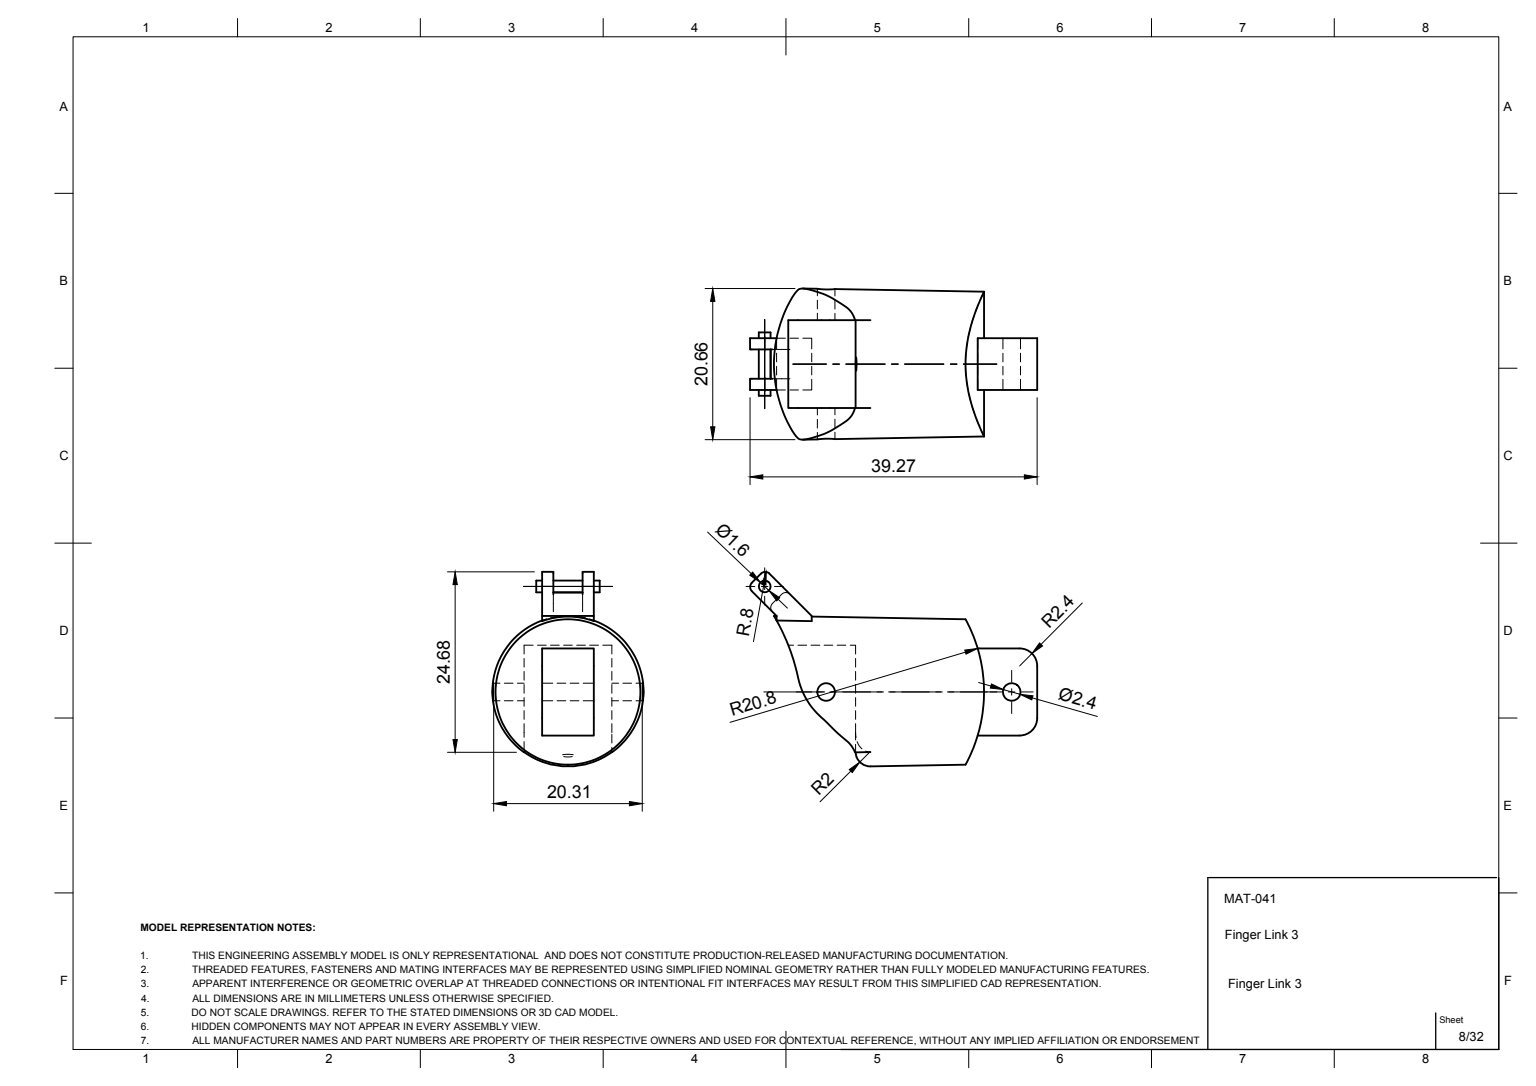
ISO-10303-21;
HEADER;
/* Generated by software containing ST-Developer
 * from STEP Tools, Inc. (www.steptools.com) 
 */

FILE_DESCRIPTION(
/* description */ ('STEP AP214'),
/* implementation_level */ '2;1');

FILE_NAME(
/* name */ 'Finger Link 3.step',
/* time_stamp */ '2026-11-14T21:57:47-08:00',
/* author */ (''),
/* organization */ (''),
/* preprocessor_version */ 'ST-DEVELOPER v20.2',
/* originating_system */ 'Autodesk Translation Framework v15.17.0.0',
/* authorisation */ '');

FILE_SCHEMA (('AUTOMOTIVE_DESIGN { 1 0 10303 214 3 1 1 }'));
ENDSEC;

DATA;
#10=MECHANICAL_DESIGN_GEOMETRIC_PRESENTATION_REPRESENTATION('',(#251),#13199);
#121=CONICAL_SURFACE('',#7376,10.4,0.0174532925199433);
#122=CONICAL_SURFACE('',#7390,10.4,0.0174532925199433);
#160=B_SPLINE_CURVE_WITH_KNOTS('',3,(#11078,#11079,#11080,#11081,#11082,
#11083,#11084,#11085,#11086,#11087,#11088,#11089,#11090,#11091,#11092,#11093,
#11094,#11095),.UNSPECIFIED.,.F.,.F.,(4,2,2,2,2,2,2,2,4),(0.904679564012803,
0.949860863856685,0.995042163700566,1.04019902886361,1.08535589402665,1.13069343457465,
1.17603097512264,1.22135607806746,1.26668118101228),.UNSPECIFIED.);
#161=B_SPLINE_CURVE_WITH_KNOTS('',3,(#11096,#11097,#11098,#11099,#11100,
#11101,#11102,#11103,#11104,#11105,#11106,#11107,#11108,#11109,#11110,#11111,
#11112,#11113,#11114),.UNSPECIFIED.,.F.,.F.,(4,2,2,2,3,2,2,2,4),(0.542677947013326,
0.588003049958145,0.633328152902964,0.678665693450959,0.724003233998953,
0.769160099161996,0.814316964325039,0.859498264168921,0.904679564012803),
 .UNSPECIFIED.);
#162=B_SPLINE_CURVE_WITH_KNOTS('',3,(#11118,#11119,#11120,#11121,#11122,
#11123,#11124,#11125,#11126,#11127,#11128,#11129,#11130,#11131,#11132,#11133,
#11134,#11135),.UNSPECIFIED.,.F.,.F.,(4,2,2,2,2,2,2,2,4),(-0.542677947013326,
-0.497352844068507,-0.452027741123688,-0.406690200575693,-0.361352660027699,
-0.316195794864656,-0.271038929701613,-0.225857629857731,-0.180676330013849),
 .UNSPECIFIED.);
#163=B_SPLINE_CURVE_WITH_KNOTS('',3,(#11139,#11140,#11141,#11142,#11143,
#11144,#11145,#11146,#11147,#11148,#11149,#11150,#11151,#11152,#11153,#11154,
#11155,#11156,#11157),.UNSPECIFIED.,.F.,.F.,(4,2,2,2,3,2,2,2,4),(-0.180676330013849,
-0.135495030169968,-0.0903137303260857,-0.0451568651630429,0.,0.0453375405479944,
0.0906750810959889,0.136000184040808,0.181325286985627),.UNSPECIFIED.);
#164=B_SPLINE_CURVE_WITH_KNOTS('',3,(#11163,#11164,#11165,#11166),
 .UNSPECIFIED.,.F.,.F.,(4,4),(0.0291654849228324,0.031266531407063),
 .UNSPECIFIED.);
#165=B_SPLINE_CURVE_WITH_KNOTS('',3,(#11168,#11169,#11170,#11171,#11172,
#11173,#11174,#11175),.UNSPECIFIED.,.F.,.F.,(4,2,2,4),(0.276435365996458,
0.375879882596353,0.487798645153617,0.537259984529731),.UNSPECIFIED.);
#166=B_SPLINE_CURVE_WITH_KNOTS('',3,(#11177,#11178,#11179,#11180),
 .UNSPECIFIED.,.F.,.F.,(4,4),(1.06524753198133,1.38156085898599),
 .UNSPECIFIED.);
#167=B_SPLINE_CURVE_WITH_KNOTS('',3,(#11182,#11183,#11184,#11185,#11186,
#11187),.UNSPECIFIED.,.F.,.F.,(4,2,4),(1.75246957687291,1.78785142251735,
1.90812306822259),.UNSPECIFIED.);
#168=B_SPLINE_CURVE_WITH_KNOTS('',3,(#11189,#11190,#11191,#11192,#11193,
#11194,#11195,#11196,#11197,#11198),.UNSPECIFIED.,.F.,.F.,(4,2,2,2,4),(5.98774864501298,
5.99007118193337,6.16584174870578,6.34161231547819,6.60463416407235),
 .UNSPECIFIED.);
#169=B_SPLINE_CURVE_WITH_KNOTS('',3,(#11200,#11201,#11202,#11203,#11204,
#11205,#11206,#11207,#11208,#11209),.UNSPECIFIED.,.F.,.F.,(4,2,2,2,4),(3.5239413534678,
3.56975642433501,3.96700634430097,4.37440770292553,4.58682119202782),
 .UNSPECIFIED.);
#170=B_SPLINE_CURVE_WITH_KNOTS('',3,(#11211,#11212,#11213,#11214,#11215,
#11216,#11217),.UNSPECIFIED.,.F.,.F.,(4,3,4),(0.0179093691038515,0.0203472114171927,
0.0227101968893206),.UNSPECIFIED.);
#171=B_SPLINE_CURVE_WITH_KNOTS('',3,(#11223,#11224,#11225,#11226,#11227,
#11228,#11229,#11230,#11231,#11232,#11233,#11234,#11235,#11236,#11237,#11238,
#11239,#11240),.UNSPECIFIED.,.F.,.F.,(4,2,2,2,2,2,2,2,4),(3.04488517957055,
3.42615346027245,3.80742174097434,4.18737194191896,4.56732214286358,4.94727660886795,
5.32723107487233,5.70850071700671,6.08977035914109),.UNSPECIFIED.);
#172=B_SPLINE_CURVE_WITH_KNOTS('',3,(#11241,#11242,#11243,#11244,#11245,
#11246,#11247,#11248,#11249,#11250,#11251,#11252,#11253,#11254,#11255,#11256,
#11257,#11258),.UNSPECIFIED.,.F.,.F.,(4,2,2,2,2,2,2,2,4),(0.,0.381269642134383,
0.762539284268766,1.14249375027314,1.52244821627752,1.90239841722213,2.28234861816675,
2.66361689886865,3.04488517957055),.UNSPECIFIED.);
#173=B_SPLINE_CURVE_WITH_KNOTS('',3,(#11262,#11263,#11264,#11265,#11266,
#11267,#11268),.UNSPECIFIED.,.F.,.F.,(4,3,4),(0.0179842259481975,0.0203472114199994,
0.0227850537330044),.UNSPECIFIED.);
#174=B_SPLINE_CURVE_WITH_KNOTS('',3,(#11270,#11271,#11272,#11273,#11274,
#11275,#11276,#11277,#11278,#11279),.UNSPECIFIED.,.F.,.F.,(4,2,2,2,4),(1.75819181671029,
1.97060530581257,2.37800666443714,2.7752565844031,2.82107165527031),
 .UNSPECIFIED.);
#175=B_SPLINE_CURVE_WITH_KNOTS('',3,(#11281,#11282,#11283,#11284,#11285,
#11286,#11287,#11288,#11289,#11290),.UNSPECIFIED.,.F.,.F.,(4,2,2,2,4),(9.36812303237173,
9.63114488096588,9.80691544773829,9.9826860145107,9.98500855143109),
 .UNSPECIFIED.);
#176=B_SPLINE_CURVE_WITH_KNOTS('',3,(#11292,#11293,#11294,#11295,#11296,
#11297),.UNSPECIFIED.,.F.,.F.,(4,2,4),(4.24121592260514,4.36148756831038,
4.39686941395482),.UNSPECIFIED.);
#177=B_SPLINE_CURVE_WITH_KNOTS('',3,(#11299,#11300,#11301,#11302),
 .UNSPECIFIED.,.F.,.F.,(4,4),(5.68043931343762,5.99675264044228),
 .UNSPECIFIED.);
#178=B_SPLINE_CURVE_WITH_KNOTS('',3,(#11304,#11305,#11306,#11307,#11308,
#11309,#11310,#11311),.UNSPECIFIED.,.F.,.F.,(4,2,2,4),(1.76236608590955,
1.81182742528566,1.92374618784292,2.02319070444282),.UNSPECIFIED.);
#179=B_SPLINE_CURVE_WITH_KNOTS('',3,(#11312,#11313,#11314,#11315),
 .UNSPECIFIED.,.F.,.F.,(4,4),(0.0094623862109046,0.0115634326876449),
 .UNSPECIFIED.);
#180=B_SPLINE_CURVE_WITH_KNOTS('',3,(#11332,#11333,#11334,#11335,#11336,
#11337,#11338,#11339,#11340,#11341,#11342,#11343,#11344),.UNSPECIFIED.,
 .F.,.F.,(4,3,2,2,2,4),(1.6015262701395,1.6049878447796,1.6729249721852,
1.74884321655348,1.83898176381711,1.95424158697802),.UNSPECIFIED.);
#181=B_SPLINE_CURVE_WITH_KNOTS('',3,(#11345,#11346,#11347,#11348,#11349,
#11350,#11351,#11352,#11353,#11354,#11355,#11356,#11357),.UNSPECIFIED.,
 .F.,.F.,(4,2,2,2,3,4),(1.25494218036839,1.36265497339682,1.4481494572272,
1.53110216280993,1.60422001043371,1.60768158507379),.UNSPECIFIED.);
#182=B_SPLINE_CURVE_WITH_KNOTS('',3,(#11359,#11360,#11361,#11362,#11363,
#11364,#11365,#11366,#11367,#11368,#11369,#11370,#11371,#11372,#11373,#11374,
#11375,#11376,#11377,#11378,#11379,#11380,#11381,#11382,#11383,#11384,#11385,
#11386,#11387,#11388,#11389,#11390,#11391,#11392,#11393,#11394,#11395,#11396,
#11397,#11398,#11399,#11400,#11401,#11402,#11403,#11404,#11405,#11406,#11407,
#11408,#11409,#11410),.UNSPECIFIED.,.T.,.F.,(4,2,2,2,2,2,2,2,2,2,2,2,2,
2,2,2,2,2,2,2,2,2,2,2,2,4),(-0.41069396663975,-0.366983311744642,-0.333124597039194,
-0.316725158605419,-0.311400724276707,-0.308795794387217,-0.307003152587989,
-0.305253095176476,-0.302970204179655,-0.299167956861605,-0.28993505003161,
-0.264304988598304,-0.228809697804181,-0.190091960609317,-0.153364093718904,
-0.124905530199035,-0.112501594518716,-0.107965577825246,-0.105609428487505,
-0.103889729748576,-0.102119162499972,-0.0996651361174354,-0.0953267397354206,
-0.0781357693656503,-0.0445945135149615,0.),.UNSPECIFIED.);
#183=B_SPLINE_CURVE_WITH_KNOTS('',3,(#11416,#11417,#11418,#11419,#11420,
#11421),.UNSPECIFIED.,.F.,.F.,(4,2,4),(-3.5239413534678,-3.17250650436905,
-2.82107165527031),.UNSPECIFIED.);
#215=SHAPE_REPRESENTATION_RELATIONSHIP('SRR','None',#13283,#233);
#233=ADVANCED_BREP_SHAPE_REPRESENTATION('',(#269),#13179);
#251=STYLED_ITEM('',(#13409),#269);
#269=MANIFOLD_SOLID_BREP('Body1',#6846);
#312=FACE_BOUND('',#2374,.T.);
#313=FACE_BOUND('',#2375,.T.);
#314=FACE_BOUND('',#2379,.T.);
#315=FACE_BOUND('',#2384,.T.);
#316=FACE_BOUND('',#2387,.T.);
#317=FACE_BOUND('',#2389,.T.);
#318=FACE_BOUND('',#2393,.T.);
#319=FACE_BOUND('',#2396,.T.);
#320=FACE_BOUND('',#2402,.T.);
#321=FACE_BOUND('',#2404,.T.);
#322=FACE_BOUND('',#2415,.T.);
#323=FACE_BOUND('',#2418,.T.);
#463=PLANE('',#7389);
#464=PLANE('',#7395);
#465=PLANE('',#7396);
#466=PLANE('',#7400);
#467=PLANE('',#7404);
#468=PLANE('',#7405);
#469=PLANE('',#7406);
#470=PLANE('',#7409);
#471=PLANE('',#7410);
#472=PLANE('',#7413);
#473=PLANE('',#7414);
#474=PLANE('',#7415);
#475=PLANE('',#7416);
#476=PLANE('',#7417);
#477=PLANE('',#7422);
#478=PLANE('',#7427);
#479=PLANE('',#7428);
#480=PLANE('',#7435);
#481=PLANE('',#7436);
#482=PLANE('',#7439);
#483=PLANE('',#7440);
#484=PLANE('',#7443);
#795=LINE('',#11052,#1313);
#796=LINE('',#11058,#1314);
#797=LINE('',#11064,#1315);
#798=LINE('',#11070,#1316);
#799=LINE('',#11076,#1317);
#800=LINE('',#11137,#1318);
#801=LINE('',#11221,#1319);
#802=LINE('',#11318,#1320);
#803=LINE('',#11321,#1321);
#804=LINE('',#11326,#1322);
#805=LINE('',#11327,#1323);
#806=LINE('',#11415,#1324);
#807=LINE('',#11423,#1325);
#808=LINE('',#11426,#1326);
#809=LINE('',#11430,#1327);
#810=LINE('',#11432,#1328);
#811=LINE('',#11434,#1329);
#812=LINE('',#11435,#1330);
#813=LINE('',#11441,#1331);
#814=LINE('',#11445,#1332);
#815=LINE('',#11449,#1333);
#816=LINE('',#11451,#1334);
#817=LINE('',#11452,#1335);
#818=LINE('',#11458,#1336);
#819=LINE('',#11463,#1337);
#820=LINE('',#11468,#1338);
#821=LINE('',#11470,#1339);
#822=LINE('',#11471,#1340);
#823=LINE('',#11475,#1341);
#824=LINE('',#11479,#1342);
#825=LINE('',#11480,#1343);
#826=LINE('',#11482,#1344);
#827=LINE('',#11486,#1345);
#828=LINE('',#11487,#1346);
#829=LINE('',#11490,#1347);
#830=LINE('',#11494,#1348);
#831=LINE('',#11497,#1349);
#832=LINE('',#11499,#1350);
#833=LINE('',#11501,#1351);
#834=LINE('',#11503,#1352);
#835=LINE('',#11504,#1353);
#836=LINE('',#11508,#1354);
#837=LINE('',#11510,#1355);
#838=LINE('',#11512,#1356);
#839=LINE('',#11513,#1357);
#840=LINE('',#11514,#1358);
#841=LINE('',#11518,#1359);
#842=LINE('',#11519,#1360);
#843=LINE('',#11520,#1361);
#844=LINE('',#11524,#1362);
#845=LINE('',#11526,#1363);
#846=LINE('',#11528,#1364);
#847=LINE('',#11529,#1365);
#848=LINE('',#11551,#1366);
#849=LINE('',#11553,#1367);
#850=LINE('',#11555,#1368);
#851=LINE('',#11556,#1369);
#852=LINE('',#11559,#1370);
#853=LINE('',#11563,#1371);
#854=LINE('',#11566,#1372);
#855=LINE('',#11567,#1373);
#856=LINE('',#11571,#1374);
#857=LINE('',#11574,#1375);
#858=LINE('',#11581,#1376);
#859=LINE('',#11583,#1377);
#1313=VECTOR('',#8618,1.2);
#1314=VECTOR('',#8625,0.800000000000001);
#1315=VECTOR('',#8632,0.800000000000001);
#1316=VECTOR('',#8639,0.800000000000001);
#1317=VECTOR('',#8646,1.2);
#1318=VECTOR('',#8649,1.2);
#1319=VECTOR('',#8658,10.4);
#1320=VECTOR('',#8663,1000.);
#1321=VECTOR('',#8666,1000.);
#1322=VECTOR('',#8671,1000.);
#1323=VECTOR('',#8672,1000.);
#1324=VECTOR('',#8681,1000.);
#1325=VECTOR('',#8682,1000.);
#1326=VECTOR('',#8685,1000.);
#1327=VECTOR('',#8688,1000.);
#1328=VECTOR('',#8689,1000.);
#1329=VECTOR('',#8690,1000.);
#1330=VECTOR('',#8691,1000.);
#1331=VECTOR('',#8698,1000.);
#1332=VECTOR('',#8701,1000.);
#1333=VECTOR('',#8706,1000.);
#1334=VECTOR('',#8707,1000.);
#1335=VECTOR('',#8708,1000.);
#1336=VECTOR('',#8717,1000.);
#1337=VECTOR('',#8724,1000.);
#1338=VECTOR('',#8731,1000.);
#1339=VECTOR('',#8732,1000.);
#1340=VECTOR('',#8733,1000.);
#1341=VECTOR('',#8736,1000.);
#1342=VECTOR('',#8739,1000.);
#1343=VECTOR('',#8740,1000.);
#1344=VECTOR('',#8741,1000.);
#1345=VECTOR('',#8746,1000.);
#1346=VECTOR('',#8747,1000.);
#1347=VECTOR('',#8750,1000.);
#1348=VECTOR('',#8755,1000.);
#1349=VECTOR('',#8758,1000.);
#1350=VECTOR('',#8759,1000.);
#1351=VECTOR('',#8760,1000.);
#1352=VECTOR('',#8761,1000.);
#1353=VECTOR('',#8762,1000.);
#1354=VECTOR('',#8765,1000.);
#1355=VECTOR('',#8766,1000.);
#1356=VECTOR('',#8767,1000.);
#1357=VECTOR('',#8768,1000.);
#1358=VECTOR('',#8769,1000.);
#1359=VECTOR('',#8772,1000.);
#1360=VECTOR('',#8773,1000.);
#1361=VECTOR('',#8774,1000.);
#1362=VECTOR('',#8777,1000.);
#1363=VECTOR('',#8778,1000.);
#1364=VECTOR('',#8779,1000.);
#1365=VECTOR('',#8780,1000.);
#1366=VECTOR('',#8819,1000.);
#1367=VECTOR('',#8820,1000.);
#1368=VECTOR('',#8821,1000.);
#1369=VECTOR('',#8822,1000.);
#1370=VECTOR('',#8825,1000.);
#1371=VECTOR('',#8830,1000.);
#1372=VECTOR('',#8833,1000.);
#1373=VECTOR('',#8834,1000.);
#1374=VECTOR('',#8839,1000.);
#1375=VECTOR('',#8844,1000.);
#1376=VECTOR('',#8857,1000.);
#1377=VECTOR('',#8860,1000.);
#1705=CYLINDRICAL_SURFACE('',#7360,1.2);
#1706=CYLINDRICAL_SURFACE('',#7363,0.800000000000001);
#1707=CYLINDRICAL_SURFACE('',#7366,0.800000000000001);
#1708=CYLINDRICAL_SURFACE('',#7369,0.800000000000001);
#1709=CYLINDRICAL_SURFACE('',#7372,1.2);
#1710=CYLINDRICAL_SURFACE('',#7374,1.2);
#1711=CYLINDRICAL_SURFACE('',#7380,16.7532667406203);
#1712=CYLINDRICAL_SURFACE('',#7382,16.7532667406203);
#1713=CYLINDRICAL_SURFACE('',#7386,28.);
#1714=CYLINDRICAL_SURFACE('',#7392,20.8);
#1715=CYLINDRICAL_SURFACE('',#7429,0.8);
#1716=CYLINDRICAL_SURFACE('',#7430,0.8);
#1717=CYLINDRICAL_SURFACE('',#7431,0.8);
#1718=CYLINDRICAL_SURFACE('',#7432,0.8);
#1719=CYLINDRICAL_SURFACE('',#7433,0.8);
#1720=CYLINDRICAL_SURFACE('',#7434,0.8);
#1721=CYLINDRICAL_SURFACE('',#7444,2.4);
#1722=CYLINDRICAL_SURFACE('',#7445,2.4);
#1723=CYLINDRICAL_SURFACE('',#7446,10.);
#1724=CYLINDRICAL_SURFACE('',#7447,10.);
#1725=CYLINDRICAL_SURFACE('',#7448,4.06015460582196);
#1726=CYLINDRICAL_SURFACE('',#7449,4.06015460582196);
#1727=CYLINDRICAL_SURFACE('',#7450,4.06015460582196);
#1728=CYLINDRICAL_SURFACE('',#7451,22.);
#1729=CYLINDRICAL_SURFACE('',#7452,22.);
#1948=FACE_OUTER_BOUND('',#2367,.T.);
#1949=FACE_OUTER_BOUND('',#2368,.T.);
#1950=FACE_OUTER_BOUND('',#2369,.T.);
#1951=FACE_OUTER_BOUND('',#2370,.T.);
#1952=FACE_OUTER_BOUND('',#2371,.T.);
#1953=FACE_OUTER_BOUND('',#2372,.T.);
#1954=FACE_OUTER_BOUND('',#2373,.T.);
#1955=FACE_OUTER_BOUND('',#2376,.T.);
#1956=FACE_OUTER_BOUND('',#2377,.T.);
#1957=FACE_OUTER_BOUND('',#2378,.T.);
#1958=FACE_OUTER_BOUND('',#2380,.T.);
#1959=FACE_OUTER_BOUND('',#2381,.T.);
#1960=FACE_OUTER_BOUND('',#2382,.T.);
#1961=FACE_OUTER_BOUND('',#2383,.T.);
#1962=FACE_OUTER_BOUND('',#2385,.T.);
#1963=FACE_OUTER_BOUND('',#2386,.T.);
#1964=FACE_OUTER_BOUND('',#2388,.T.);
#1965=FACE_OUTER_BOUND('',#2390,.T.);
#1966=FACE_OUTER_BOUND('',#2391,.T.);
#1967=FACE_OUTER_BOUND('',#2392,.T.);
#1968=FACE_OUTER_BOUND('',#2394,.T.);
#1969=FACE_OUTER_BOUND('',#2395,.T.);
#1970=FACE_OUTER_BOUND('',#2397,.T.);
#1971=FACE_OUTER_BOUND('',#2398,.T.);
#1972=FACE_OUTER_BOUND('',#2399,.T.);
#1973=FACE_OUTER_BOUND('',#2400,.T.);
#1974=FACE_OUTER_BOUND('',#2401,.T.);
#1975=FACE_OUTER_BOUND('',#2403,.T.);
#1976=FACE_OUTER_BOUND('',#2405,.T.);
#1977=FACE_OUTER_BOUND('',#2406,.T.);
#1978=FACE_OUTER_BOUND('',#2407,.T.);
#1979=FACE_OUTER_BOUND('',#2408,.T.);
#1980=FACE_OUTER_BOUND('',#2409,.T.);
#1981=FACE_OUTER_BOUND('',#2410,.T.);
#1982=FACE_OUTER_BOUND('',#2411,.T.);
#1983=FACE_OUTER_BOUND('',#2412,.T.);
#1984=FACE_OUTER_BOUND('',#2413,.T.);
#1985=FACE_OUTER_BOUND('',#2414,.T.);
#1986=FACE_OUTER_BOUND('',#2416,.T.);
#1987=FACE_OUTER_BOUND('',#2417,.T.);
#1988=FACE_OUTER_BOUND('',#2419,.T.);
#1989=FACE_OUTER_BOUND('',#2420,.T.);
#1990=FACE_OUTER_BOUND('',#2421,.T.);
#1991=FACE_OUTER_BOUND('',#2422,.T.);
#1992=FACE_OUTER_BOUND('',#2423,.T.);
#1993=FACE_OUTER_BOUND('',#2424,.T.);
#1994=FACE_OUTER_BOUND('',#2425,.T.);
#1995=FACE_OUTER_BOUND('',#2426,.T.);
#1996=FACE_OUTER_BOUND('',#2427,.T.);
#1997=FACE_OUTER_BOUND('',#2428,.T.);
#2367=EDGE_LOOP('',(#5286,#5287,#5288,#5289));
#2368=EDGE_LOOP('',(#5290,#5291,#5292,#5293));
#2369=EDGE_LOOP('',(#5294,#5295,#5296,#5297));
#2370=EDGE_LOOP('',(#5298,#5299,#5300,#5301));
#2371=EDGE_LOOP('',(#5302,#5303,#5304,#5305,#5306));
#2372=EDGE_LOOP('',(#5307,#5308,#5309,#5310,#5311));
#2373=EDGE_LOOP('',(#5312,#5313,#5314,#5315,#5316,#5317,#5318,#5319,#5320,
#5321,#5322,#5323,#5324,#5325,#5326,#5327,#5328,#5329,#5330,#5331,#5332));
#2374=EDGE_LOOP('',(#5333,#5334));
#2375=EDGE_LOOP('',(#5335,#5336));
#2376=EDGE_LOOP('',(#5337,#5338,#5339,#5340));
#2377=EDGE_LOOP('',(#5341,#5342,#5343,#5344));
#2378=EDGE_LOOP('',(#5345,#5346,#5347,#5348));
#2379=EDGE_LOOP('',(#5349));
#2380=EDGE_LOOP('',(#5350,#5351,#5352,#5353,#5354,#5355,#5356,#5357));
#2381=EDGE_LOOP('',(#5358,#5359,#5360,#5361));
#2382=EDGE_LOOP('',(#5362,#5363));
#2383=EDGE_LOOP('',(#5364,#5365));
#2384=EDGE_LOOP('',(#5366,#5367,#5368,#5369));
#2385=EDGE_LOOP('',(#5370,#5371,#5372,#5373));
#2386=EDGE_LOOP('',(#5374,#5375,#5376,#5377,#5378,#5379,#5380,#5381,#5382));
#2387=EDGE_LOOP('',(#5383));
#2388=EDGE_LOOP('',(#5384,#5385,#5386,#5387,#5388,#5389,#5390,#5391,#5392));
#2389=EDGE_LOOP('',(#5393));
#2390=EDGE_LOOP('',(#5394,#5395,#5396,#5397));
#2391=EDGE_LOOP('',(#5398,#5399,#5400,#5401));
#2392=EDGE_LOOP('',(#5402,#5403,#5404,#5405,#5406,#5407,#5408,#5409));
#2393=EDGE_LOOP('',(#5410));
#2394=EDGE_LOOP('',(#5411,#5412,#5413,#5414,#5415));
#2395=EDGE_LOOP('',(#5416,#5417,#5418,#5419,#5420,#5421,#5422,#5423));
#2396=EDGE_LOOP('',(#5424));
#2397=EDGE_LOOP('',(#5425,#5426,#5427,#5428,#5429,#5430,#5431,#5432));
#2398=EDGE_LOOP('',(#5433,#5434,#5435,#5436,#5437,#5438,#5439,#5440));
#2399=EDGE_LOOP('',(#5441,#5442,#5443,#5444));
#2400=EDGE_LOOP('',(#5445,#5446,#5447,#5448));
#2401=EDGE_LOOP('',(#5449,#5450,#5451,#5452,#5453,#5454,#5455,#5456));
#2402=EDGE_LOOP('',(#5457));
#2403=EDGE_LOOP('',(#5458,#5459,#5460,#5461,#5462,#5463,#5464,#5465));
#2404=EDGE_LOOP('',(#5466));
#2405=EDGE_LOOP('',(#5467));
#2406=EDGE_LOOP('',(#5468));
#2407=EDGE_LOOP('',(#5469,#5470,#5471,#5472));
#2408=EDGE_LOOP('',(#5473,#5474,#5475,#5476));
#2409=EDGE_LOOP('',(#5477,#5478,#5479,#5480));
#2410=EDGE_LOOP('',(#5481,#5482,#5483,#5484));
#2411=EDGE_LOOP('',(#5485,#5486,#5487,#5488));
#2412=EDGE_LOOP('',(#5489,#5490,#5491,#5492));
#2413=EDGE_LOOP('',(#5493,#5494,#5495,#5496));
#2414=EDGE_LOOP('',(#5497,#5498,#5499,#5500,#5501,#5502));
#2415=EDGE_LOOP('',(#5503));
#2416=EDGE_LOOP('',(#5504,#5505,#5506,#5507));
#2417=EDGE_LOOP('',(#5508,#5509,#5510,#5511,#5512,#5513));
#2418=EDGE_LOOP('',(#5514));
#2419=EDGE_LOOP('',(#5515,#5516,#5517,#5518));
#2420=EDGE_LOOP('',(#5519,#5520,#5521,#5522));
#2421=EDGE_LOOP('',(#5523,#5524,#5525,#5526));
#2422=EDGE_LOOP('',(#5527,#5528,#5529,#5530));
#2423=EDGE_LOOP('',(#5531,#5532,#5533,#5534));
#2424=EDGE_LOOP('',(#5535));
#2425=EDGE_LOOP('',(#5536,#5537,#5538));
#2426=EDGE_LOOP('',(#5539,#5540,#5541));
#2427=EDGE_LOOP('',(#5542,#5543,#5544,#5545));
#2428=EDGE_LOOP('',(#5546,#5547,#5548,#5549));
#2818=CIRCLE('',#7361,1.2);
#2819=CIRCLE('',#7362,1.2);
#2820=CIRCLE('',#7364,0.800000000000001);
#2821=CIRCLE('',#7365,0.800000000000001);
#2822=CIRCLE('',#7367,0.800000000000001);
#2823=CIRCLE('',#7368,0.800000000000001);
#2824=CIRCLE('',#7370,0.800000000000001);
#2825=CIRCLE('',#7371,0.800000000000001);
#2826=CIRCLE('',#7373,1.2);
#2827=CIRCLE('',#7375,1.2);
#2828=CIRCLE('',#7377,10.169681257704);
#2829=CIRCLE('',#7378,10.3099206524828);
#2830=CIRCLE('',#7379,10.3099206524828);
#2831=CIRCLE('',#7381,16.7532667406203);
#2832=CIRCLE('',#7383,16.7532667406203);
#2833=CIRCLE('',#7385,8.16998586739121);
#2834=CIRCLE('',#7387,28.);
#2835=CIRCLE('',#7388,28.);
#2836=CIRCLE('',#7391,10.3937049641382);
#2837=CIRCLE('',#7393,20.8);
#2838=CIRCLE('',#7394,20.8);
#2839=CIRCLE('',#7397,4.06015460582196);
#2840=CIRCLE('',#7398,22.);
#2841=CIRCLE('',#7399,10.);
#2842=CIRCLE('',#7401,22.);
#2843=CIRCLE('',#7402,4.06015460582196);
#2844=CIRCLE('',#7403,10.);
#2845=CIRCLE('',#7407,0.8);
#2846=CIRCLE('',#7408,0.8);
#2847=CIRCLE('',#7411,0.8);
#2848=CIRCLE('',#7412,0.8);
#2849=CIRCLE('',#7418,0.8);
#2850=CIRCLE('',#7419,0.8);
#2851=CIRCLE('',#7420,0.8);
#2852=CIRCLE('',#7421,0.8);
#2853=CIRCLE('',#7423,0.8);
#2854=CIRCLE('',#7424,0.8);
#2855=CIRCLE('',#7425,0.8);
#2856=CIRCLE('',#7426,0.8);
#2857=CIRCLE('',#7437,2.4);
#2858=CIRCLE('',#7438,2.4);
#2859=CIRCLE('',#7441,2.4);
#2860=CIRCLE('',#7442,2.4);
#3230=VERTEX_POINT('',#11049);
#3231=VERTEX_POINT('',#11051);
#3232=VERTEX_POINT('',#11055);
#3233=VERTEX_POINT('',#11057);
#3234=VERTEX_POINT('',#11061);
#3235=VERTEX_POINT('',#11063);
#3236=VERTEX_POINT('',#11067);
#3237=VERTEX_POINT('',#11069);
#3238=VERTEX_POINT('',#11073);
#3239=VERTEX_POINT('',#11075);
#3240=VERTEX_POINT('',#11077);
#3241=VERTEX_POINT('',#11116);
#3242=VERTEX_POINT('',#11117);
#3243=VERTEX_POINT('',#11136);
#3244=VERTEX_POINT('',#11159);
#3245=VERTEX_POINT('',#11160);
#3246=VERTEX_POINT('',#11162);
#3247=VERTEX_POINT('',#11167);
#3248=VERTEX_POINT('',#11176);
#3249=VERTEX_POINT('',#11181);
#3250=VERTEX_POINT('',#11188);
#3251=VERTEX_POINT('',#11199);
#3252=VERTEX_POINT('',#11210);
#3253=VERTEX_POINT('',#11218);
#3254=VERTEX_POINT('',#11220);
#3255=VERTEX_POINT('',#11222);
#3256=VERTEX_POINT('',#11259);
#3257=VERTEX_POINT('',#11261);
#3258=VERTEX_POINT('',#11269);
#3259=VERTEX_POINT('',#11280);
#3260=VERTEX_POINT('',#11291);
#3261=VERTEX_POINT('',#11298);
#3262=VERTEX_POINT('',#11303);
#3263=VERTEX_POINT('',#11317);
#3264=VERTEX_POINT('',#11319);
#3265=VERTEX_POINT('',#11323);
#3266=VERTEX_POINT('',#11324);
#3267=VERTEX_POINT('',#11329);
#3268=VERTEX_POINT('',#11330);
#3269=VERTEX_POINT('',#11358);
#3270=VERTEX_POINT('',#11412);
#3271=VERTEX_POINT('',#11413);
#3272=VERTEX_POINT('',#11422);
#3273=VERTEX_POINT('',#11424);
#3274=VERTEX_POINT('',#11428);
#3275=VERTEX_POINT('',#11429);
#3276=VERTEX_POINT('',#11431);
#3277=VERTEX_POINT('',#11433);
#3278=VERTEX_POINT('',#11439);
#3279=VERTEX_POINT('',#11440);
#3280=VERTEX_POINT('',#11442);
#3281=VERTEX_POINT('',#11444);
#3282=VERTEX_POINT('',#11448);
#3283=VERTEX_POINT('',#11450);
#3284=VERTEX_POINT('',#11454);
#3285=VERTEX_POINT('',#11460);
#3286=VERTEX_POINT('',#11467);
#3287=VERTEX_POINT('',#11469);
#3288=VERTEX_POINT('',#11473);
#3289=VERTEX_POINT('',#11474);
#3290=VERTEX_POINT('',#11476);
#3291=VERTEX_POINT('',#11478);
#3292=VERTEX_POINT('',#11481);
#3293=VERTEX_POINT('',#11485);
#3294=VERTEX_POINT('',#11489);
#3295=VERTEX_POINT('',#11492);
#3296=VERTEX_POINT('',#11496);
#3297=VERTEX_POINT('',#11498);
#3298=VERTEX_POINT('',#11500);
#3299=VERTEX_POINT('',#11502);
#3300=VERTEX_POINT('',#11506);
#3301=VERTEX_POINT('',#11507);
#3302=VERTEX_POINT('',#11509);
#3303=VERTEX_POINT('',#11511);
#3304=VERTEX_POINT('',#11516);
#3305=VERTEX_POINT('',#11517);
#3306=VERTEX_POINT('',#11522);
#3307=VERTEX_POINT('',#11523);
#3308=VERTEX_POINT('',#11525);
#3309=VERTEX_POINT('',#11527);
#3310=VERTEX_POINT('',#11549);
#3311=VERTEX_POINT('',#11550);
#3312=VERTEX_POINT('',#11552);
#3313=VERTEX_POINT('',#11554);
#3314=VERTEX_POINT('',#11558);
#3315=VERTEX_POINT('',#11561);
#3316=VERTEX_POINT('',#11565);
#3317=VERTEX_POINT('',#11570);
#3980=EDGE_CURVE('',#3230,#3230,#2818,.T.);
#3981=EDGE_CURVE('',#3230,#3231,#795,.T.);
#3982=EDGE_CURVE('',#3231,#3231,#2819,.T.);
#3983=EDGE_CURVE('',#3232,#3232,#2820,.T.);
#3984=EDGE_CURVE('',#3232,#3233,#796,.T.);
#3985=EDGE_CURVE('',#3233,#3233,#2821,.T.);
#3986=EDGE_CURVE('',#3234,#3234,#2822,.T.);
#3987=EDGE_CURVE('',#3234,#3235,#797,.T.);
#3988=EDGE_CURVE('',#3235,#3235,#2823,.T.);
#3989=EDGE_CURVE('',#3236,#3236,#2824,.T.);
#3990=EDGE_CURVE('',#3236,#3237,#798,.T.);
#3991=EDGE_CURVE('',#3237,#3237,#2825,.T.);
#3992=EDGE_CURVE('',#3238,#3238,#2826,.T.);
#3993=EDGE_CURVE('',#3238,#3239,#799,.T.);
#3994=EDGE_CURVE('',#3239,#3240,#160,.T.);
#3995=EDGE_CURVE('',#3240,#3239,#161,.T.);
#3996=EDGE_CURVE('',#3241,#3242,#162,.T.);
#3997=EDGE_CURVE('',#3242,#3243,#800,.T.);
#3998=EDGE_CURVE('',#3243,#3243,#2827,.T.);
#3999=EDGE_CURVE('',#3242,#3241,#163,.T.);
#4000=EDGE_CURVE('',#3244,#3245,#2828,.T.);
#4001=EDGE_CURVE('',#3246,#3245,#164,.T.);
#4002=EDGE_CURVE('',#3247,#3246,#165,.T.);
#4003=EDGE_CURVE('',#3247,#3248,#166,.T.);
#4004=EDGE_CURVE('',#3249,#3248,#167,.T.);
#4005=EDGE_CURVE('',#3249,#3250,#168,.T.);
#4006=EDGE_CURVE('',#3251,#3250,#169,.T.);
#4007=EDGE_CURVE('',#3251,#3252,#170,.T.);
#4008=EDGE_CURVE('',#3252,#3253,#2829,.T.);
#4009=EDGE_CURVE('',#3253,#3254,#801,.T.);
#4010=EDGE_CURVE('',#3254,#3255,#171,.T.);
#4011=EDGE_CURVE('',#3255,#3254,#172,.T.);
#4012=EDGE_CURVE('',#3253,#3256,#2830,.T.);
#4013=EDGE_CURVE('',#3256,#3257,#173,.T.);
#4014=EDGE_CURVE('',#3258,#3257,#174,.T.);
#4015=EDGE_CURVE('',#3258,#3259,#175,.T.);
#4016=EDGE_CURVE('',#3260,#3259,#176,.T.);
#4017=EDGE_CURVE('',#3260,#3261,#177,.T.);
#4018=EDGE_CURVE('',#3262,#3261,#178,.T.);
#4019=EDGE_CURVE('',#3244,#3262,#179,.T.);
#4020=EDGE_CURVE('',#3248,#3263,#802,.T.);
#4021=EDGE_CURVE('',#3264,#3263,#2831,.T.);
#4022=EDGE_CURVE('',#3264,#3249,#803,.T.);
#4023=EDGE_CURVE('',#3265,#3266,#2832,.T.);
#4024=EDGE_CURVE('',#3265,#3260,#804,.T.);
#4025=EDGE_CURVE('',#3259,#3266,#805,.T.);
#4026=EDGE_CURVE('',#3267,#3268,#2833,.T.);
#4027=EDGE_CURVE('',#3245,#3267,#180,.T.);
#4028=EDGE_CURVE('',#3268,#3244,#181,.T.);
#4029=EDGE_CURVE('',#3269,#3269,#182,.T.);
#4030=EDGE_CURVE('',#3270,#3271,#2834,.T.);
#4031=EDGE_CURVE('',#3271,#3258,#806,.T.);
#4032=EDGE_CURVE('',#3257,#3251,#183,.T.);
#4033=EDGE_CURVE('',#3250,#3272,#807,.T.);
#4034=EDGE_CURVE('',#3272,#3273,#2835,.T.);
#4035=EDGE_CURVE('',#3270,#3273,#808,.T.);
#4036=EDGE_CURVE('',#3274,#3275,#809,.T.);
#4037=EDGE_CURVE('',#3275,#3276,#810,.T.);
#4038=EDGE_CURVE('',#3277,#3276,#811,.T.);
#4039=EDGE_CURVE('',#3277,#3274,#812,.T.);
#4040=EDGE_CURVE('',#3257,#3251,#2836,.T.);
#4041=EDGE_CURVE('',#3278,#3279,#813,.T.);
#4042=EDGE_CURVE('',#3280,#3278,#2837,.T.);
#4043=EDGE_CURVE('',#3281,#3280,#814,.T.);
#4044=EDGE_CURVE('',#3279,#3281,#2838,.T.);
#4045=EDGE_CURVE('',#3268,#3282,#815,.T.);
#4046=EDGE_CURVE('',#3283,#3282,#816,.T.);
#4047=EDGE_CURVE('',#3267,#3283,#817,.T.);
#4048=EDGE_CURVE('',#3262,#3284,#2839,.T.);
#4049=EDGE_CURVE('',#3284,#3265,#2840,.T.);
#4050=EDGE_CURVE('',#3266,#3271,#2841,.T.);
#4051=EDGE_CURVE('',#3282,#3270,#818,.T.);
#4052=EDGE_CURVE('',#3263,#3285,#2842,.T.);
#4053=EDGE_CURVE('',#3285,#3246,#2843,.T.);
#4054=EDGE_CURVE('',#3273,#3283,#819,.T.);
#4055=EDGE_CURVE('',#3272,#3264,#2844,.T.);
#4056=EDGE_CURVE('',#3257,#3286,#820,.T.);
#4057=EDGE_CURVE('',#3286,#3287,#821,.T.);
#4058=EDGE_CURVE('',#3251,#3287,#822,.T.);
#4059=EDGE_CURVE('',#3288,#3289,#823,.T.);
#4060=EDGE_CURVE('',#3288,#3290,#2845,.T.);
#4061=EDGE_CURVE('',#3290,#3291,#824,.T.);
#4062=EDGE_CURVE('',#3252,#3291,#825,.T.);
#4063=EDGE_CURVE('',#3292,#3287,#826,.T.);
#4064=EDGE_CURVE('',#3292,#3289,#2846,.T.);
#4065=EDGE_CURVE('',#3291,#3293,#827,.T.);
#4066=EDGE_CURVE('',#3256,#3293,#828,.T.);
#4067=EDGE_CURVE('',#3294,#3293,#829,.T.);
#4068=EDGE_CURVE('',#3294,#3275,#2847,.T.);
#4069=EDGE_CURVE('',#3274,#3295,#2848,.T.);
#4070=EDGE_CURVE('',#3295,#3286,#830,.T.);
#4071=EDGE_CURVE('',#3295,#3296,#831,.T.);
#4072=EDGE_CURVE('',#3296,#3297,#832,.T.);
#4073=EDGE_CURVE('',#3297,#3298,#833,.T.);
#4074=EDGE_CURVE('',#3298,#3299,#834,.T.);
#4075=EDGE_CURVE('',#3299,#3292,#835,.T.);
#4076=EDGE_CURVE('',#3300,#3301,#836,.T.);
#4077=EDGE_CURVE('',#3300,#3302,#837,.T.);
#4078=EDGE_CURVE('',#3303,#3302,#838,.T.);
#4079=EDGE_CURVE('',#3303,#3294,#839,.T.);
#4080=EDGE_CURVE('',#3290,#3301,#840,.T.);
#4081=EDGE_CURVE('',#3304,#3305,#841,.T.);
#4082=EDGE_CURVE('',#3304,#3288,#842,.T.);
#4083=EDGE_CURVE('',#3289,#3305,#843,.T.);
#4084=EDGE_CURVE('',#3306,#3307,#844,.T.);
#4085=EDGE_CURVE('',#3307,#3308,#845,.T.);
#4086=EDGE_CURVE('',#3309,#3308,#846,.T.);
#4087=EDGE_CURVE('',#3309,#3306,#847,.T.);
#4088=EDGE_CURVE('',#3276,#3303,#2849,.T.);
#4089=EDGE_CURVE('',#3302,#3307,#2850,.T.);
#4090=EDGE_CURVE('',#3306,#3297,#2851,.T.);
#4091=EDGE_CURVE('',#3296,#3277,#2852,.T.);
#4092=EDGE_CURVE('',#3301,#3304,#2853,.T.);
#4093=EDGE_CURVE('',#3305,#3299,#2854,.T.);
#4094=EDGE_CURVE('',#3298,#3309,#2855,.T.);
#4095=EDGE_CURVE('',#3308,#3300,#2856,.T.);
#4096=EDGE_CURVE('',#3310,#3311,#848,.T.);
#4097=EDGE_CURVE('',#3311,#3312,#849,.T.);
#4098=EDGE_CURVE('',#3312,#3313,#850,.T.);
#4099=EDGE_CURVE('',#3313,#3310,#851,.T.);
#4100=EDGE_CURVE('',#3278,#3314,#852,.T.);
#4101=EDGE_CURVE('',#3314,#3311,#2857,.T.);
#4102=EDGE_CURVE('',#3310,#3315,#2858,.T.);
#4103=EDGE_CURVE('',#3280,#3315,#853,.T.);
#4104=EDGE_CURVE('',#3279,#3316,#854,.T.);
#4105=EDGE_CURVE('',#3316,#3314,#855,.T.);
#4106=EDGE_CURVE('',#3312,#3316,#2859,.T.);
#4107=EDGE_CURVE('',#3281,#3317,#856,.T.);
#4108=EDGE_CURVE('',#3317,#3313,#2860,.T.);
#4109=EDGE_CURVE('',#3315,#3317,#857,.T.);
#4110=EDGE_CURVE('',#3261,#3284,#858,.T.);
#4111=EDGE_CURVE('',#3285,#3247,#859,.T.);
#5286=ORIENTED_EDGE('',*,*,#3980,.T.);
#5287=ORIENTED_EDGE('',*,*,#3981,.T.);
#5288=ORIENTED_EDGE('',*,*,#3982,.T.);
#5289=ORIENTED_EDGE('',*,*,#3981,.F.);
#5290=ORIENTED_EDGE('',*,*,#3983,.T.);
#5291=ORIENTED_EDGE('',*,*,#3984,.T.);
#5292=ORIENTED_EDGE('',*,*,#3985,.T.);
#5293=ORIENTED_EDGE('',*,*,#3984,.F.);
#5294=ORIENTED_EDGE('',*,*,#3986,.T.);
#5295=ORIENTED_EDGE('',*,*,#3987,.T.);
#5296=ORIENTED_EDGE('',*,*,#3988,.F.);
#5297=ORIENTED_EDGE('',*,*,#3987,.F.);
#5298=ORIENTED_EDGE('',*,*,#3989,.T.);
#5299=ORIENTED_EDGE('',*,*,#3990,.T.);
#5300=ORIENTED_EDGE('',*,*,#3991,.T.);
#5301=ORIENTED_EDGE('',*,*,#3990,.F.);
#5302=ORIENTED_EDGE('',*,*,#3992,.F.);
#5303=ORIENTED_EDGE('',*,*,#3993,.T.);
#5304=ORIENTED_EDGE('',*,*,#3994,.T.);
#5305=ORIENTED_EDGE('',*,*,#3995,.T.);
#5306=ORIENTED_EDGE('',*,*,#3993,.F.);
#5307=ORIENTED_EDGE('',*,*,#3996,.T.);
#5308=ORIENTED_EDGE('',*,*,#3997,.T.);
#5309=ORIENTED_EDGE('',*,*,#3998,.F.);
#5310=ORIENTED_EDGE('',*,*,#3997,.F.);
#5311=ORIENTED_EDGE('',*,*,#3999,.T.);
#5312=ORIENTED_EDGE('',*,*,#4000,.T.);
#5313=ORIENTED_EDGE('',*,*,#4001,.F.);
#5314=ORIENTED_EDGE('',*,*,#4002,.F.);
#5315=ORIENTED_EDGE('',*,*,#4003,.T.);
#5316=ORIENTED_EDGE('',*,*,#4004,.F.);
#5317=ORIENTED_EDGE('',*,*,#4005,.T.);
#5318=ORIENTED_EDGE('',*,*,#4006,.F.);
#5319=ORIENTED_EDGE('',*,*,#4007,.T.);
#5320=ORIENTED_EDGE('',*,*,#4008,.T.);
#5321=ORIENTED_EDGE('',*,*,#4009,.T.);
#5322=ORIENTED_EDGE('',*,*,#4010,.T.);
#5323=ORIENTED_EDGE('',*,*,#4011,.T.);
#5324=ORIENTED_EDGE('',*,*,#4009,.F.);
#5325=ORIENTED_EDGE('',*,*,#4012,.T.);
#5326=ORIENTED_EDGE('',*,*,#4013,.T.);
#5327=ORIENTED_EDGE('',*,*,#4014,.F.);
#5328=ORIENTED_EDGE('',*,*,#4015,.T.);
#5329=ORIENTED_EDGE('',*,*,#4016,.F.);
#5330=ORIENTED_EDGE('',*,*,#4017,.T.);
#5331=ORIENTED_EDGE('',*,*,#4018,.F.);
#5332=ORIENTED_EDGE('',*,*,#4019,.F.);
#5333=ORIENTED_EDGE('',*,*,#3996,.F.);
#5334=ORIENTED_EDGE('',*,*,#3999,.F.);
#5335=ORIENTED_EDGE('',*,*,#3995,.F.);
#5336=ORIENTED_EDGE('',*,*,#3994,.F.);
#5337=ORIENTED_EDGE('',*,*,#4004,.T.);
#5338=ORIENTED_EDGE('',*,*,#4020,.T.);
#5339=ORIENTED_EDGE('',*,*,#4021,.F.);
#5340=ORIENTED_EDGE('',*,*,#4022,.T.);
#5341=ORIENTED_EDGE('',*,*,#4023,.F.);
#5342=ORIENTED_EDGE('',*,*,#4024,.T.);
#5343=ORIENTED_EDGE('',*,*,#4016,.T.);
#5344=ORIENTED_EDGE('',*,*,#4025,.T.);
#5345=ORIENTED_EDGE('',*,*,#4026,.F.);
#5346=ORIENTED_EDGE('',*,*,#4027,.F.);
#5347=ORIENTED_EDGE('',*,*,#4000,.F.);
#5348=ORIENTED_EDGE('',*,*,#4028,.F.);
#5349=ORIENTED_EDGE('',*,*,#4029,.T.);
#5350=ORIENTED_EDGE('',*,*,#4030,.T.);
#5351=ORIENTED_EDGE('',*,*,#4031,.T.);
#5352=ORIENTED_EDGE('',*,*,#4014,.T.);
#5353=ORIENTED_EDGE('',*,*,#4032,.T.);
#5354=ORIENTED_EDGE('',*,*,#4006,.T.);
#5355=ORIENTED_EDGE('',*,*,#4033,.T.);
#5356=ORIENTED_EDGE('',*,*,#4034,.T.);
#5357=ORIENTED_EDGE('',*,*,#4035,.F.);
#5358=ORIENTED_EDGE('',*,*,#4036,.T.);
#5359=ORIENTED_EDGE('',*,*,#4037,.T.);
#5360=ORIENTED_EDGE('',*,*,#4038,.F.);
#5361=ORIENTED_EDGE('',*,*,#4039,.T.);
#5362=ORIENTED_EDGE('',*,*,#4040,.T.);
#5363=ORIENTED_EDGE('',*,*,#4032,.F.);
#5364=ORIENTED_EDGE('',*,*,#4011,.F.);
#5365=ORIENTED_EDGE('',*,*,#4010,.F.);
#5366=ORIENTED_EDGE('',*,*,#4041,.F.);
#5367=ORIENTED_EDGE('',*,*,#4042,.F.);
#5368=ORIENTED_EDGE('',*,*,#4043,.F.);
#5369=ORIENTED_EDGE('',*,*,#4044,.F.);
#5370=ORIENTED_EDGE('',*,*,#4026,.T.);
#5371=ORIENTED_EDGE('',*,*,#4045,.T.);
#5372=ORIENTED_EDGE('',*,*,#4046,.F.);
#5373=ORIENTED_EDGE('',*,*,#4047,.F.);
#5374=ORIENTED_EDGE('',*,*,#4048,.T.);
#5375=ORIENTED_EDGE('',*,*,#4049,.T.);
#5376=ORIENTED_EDGE('',*,*,#4023,.T.);
#5377=ORIENTED_EDGE('',*,*,#4050,.T.);
#5378=ORIENTED_EDGE('',*,*,#4030,.F.);
#5379=ORIENTED_EDGE('',*,*,#4051,.F.);
#5380=ORIENTED_EDGE('',*,*,#4045,.F.);
#5381=ORIENTED_EDGE('',*,*,#4028,.T.);
#5382=ORIENTED_EDGE('',*,*,#4019,.T.);
#5383=ORIENTED_EDGE('',*,*,#3992,.T.);
#5384=ORIENTED_EDGE('',*,*,#4021,.T.);
#5385=ORIENTED_EDGE('',*,*,#4052,.T.);
#5386=ORIENTED_EDGE('',*,*,#4053,.T.);
#5387=ORIENTED_EDGE('',*,*,#4001,.T.);
#5388=ORIENTED_EDGE('',*,*,#4027,.T.);
#5389=ORIENTED_EDGE('',*,*,#4047,.T.);
#5390=ORIENTED_EDGE('',*,*,#4054,.F.);
#5391=ORIENTED_EDGE('',*,*,#4034,.F.);
#5392=ORIENTED_EDGE('',*,*,#4055,.T.);
#5393=ORIENTED_EDGE('',*,*,#3998,.T.);
#5394=ORIENTED_EDGE('',*,*,#4035,.T.);
#5395=ORIENTED_EDGE('',*,*,#4054,.T.);
#5396=ORIENTED_EDGE('',*,*,#4046,.T.);
#5397=ORIENTED_EDGE('',*,*,#4051,.T.);
#5398=ORIENTED_EDGE('',*,*,#4040,.F.);
#5399=ORIENTED_EDGE('',*,*,#4056,.T.);
#5400=ORIENTED_EDGE('',*,*,#4057,.T.);
#5401=ORIENTED_EDGE('',*,*,#4058,.F.);
#5402=ORIENTED_EDGE('',*,*,#4059,.F.);
#5403=ORIENTED_EDGE('',*,*,#4060,.T.);
#5404=ORIENTED_EDGE('',*,*,#4061,.T.);
#5405=ORIENTED_EDGE('',*,*,#4062,.F.);
#5406=ORIENTED_EDGE('',*,*,#4007,.F.);
#5407=ORIENTED_EDGE('',*,*,#4058,.T.);
#5408=ORIENTED_EDGE('',*,*,#4063,.F.);
#5409=ORIENTED_EDGE('',*,*,#4064,.T.);
#5410=ORIENTED_EDGE('',*,*,#3985,.F.);
#5411=ORIENTED_EDGE('',*,*,#4008,.F.);
#5412=ORIENTED_EDGE('',*,*,#4062,.T.);
#5413=ORIENTED_EDGE('',*,*,#4065,.T.);
#5414=ORIENTED_EDGE('',*,*,#4066,.F.);
#5415=ORIENTED_EDGE('',*,*,#4012,.F.);
#5416=ORIENTED_EDGE('',*,*,#4067,.F.);
#5417=ORIENTED_EDGE('',*,*,#4068,.T.);
#5418=ORIENTED_EDGE('',*,*,#4036,.F.);
#5419=ORIENTED_EDGE('',*,*,#4069,.T.);
#5420=ORIENTED_EDGE('',*,*,#4070,.T.);
#5421=ORIENTED_EDGE('',*,*,#4056,.F.);
#5422=ORIENTED_EDGE('',*,*,#4013,.F.);
#5423=ORIENTED_EDGE('',*,*,#4066,.T.);
#5424=ORIENTED_EDGE('',*,*,#3986,.F.);
#5425=ORIENTED_EDGE('',*,*,#4070,.F.);
#5426=ORIENTED_EDGE('',*,*,#4071,.T.);
#5427=ORIENTED_EDGE('',*,*,#4072,.T.);
#5428=ORIENTED_EDGE('',*,*,#4073,.T.);
#5429=ORIENTED_EDGE('',*,*,#4074,.T.);
#5430=ORIENTED_EDGE('',*,*,#4075,.T.);
#5431=ORIENTED_EDGE('',*,*,#4063,.T.);
#5432=ORIENTED_EDGE('',*,*,#4057,.F.);
#5433=ORIENTED_EDGE('',*,*,#4076,.F.);
#5434=ORIENTED_EDGE('',*,*,#4077,.T.);
#5435=ORIENTED_EDGE('',*,*,#4078,.F.);
#5436=ORIENTED_EDGE('',*,*,#4079,.T.);
#5437=ORIENTED_EDGE('',*,*,#4067,.T.);
#5438=ORIENTED_EDGE('',*,*,#4065,.F.);
#5439=ORIENTED_EDGE('',*,*,#4061,.F.);
#5440=ORIENTED_EDGE('',*,*,#4080,.T.);
#5441=ORIENTED_EDGE('',*,*,#4081,.F.);
#5442=ORIENTED_EDGE('',*,*,#4082,.T.);
#5443=ORIENTED_EDGE('',*,*,#4059,.T.);
#5444=ORIENTED_EDGE('',*,*,#4083,.T.);
#5445=ORIENTED_EDGE('',*,*,#4084,.T.);
#5446=ORIENTED_EDGE('',*,*,#4085,.T.);
#5447=ORIENTED_EDGE('',*,*,#4086,.F.);
#5448=ORIENTED_EDGE('',*,*,#4087,.T.);
#5449=ORIENTED_EDGE('',*,*,#4038,.T.);
#5450=ORIENTED_EDGE('',*,*,#4088,.T.);
#5451=ORIENTED_EDGE('',*,*,#4078,.T.);
#5452=ORIENTED_EDGE('',*,*,#4089,.T.);
#5453=ORIENTED_EDGE('',*,*,#4084,.F.);
#5454=ORIENTED_EDGE('',*,*,#4090,.T.);
#5455=ORIENTED_EDGE('',*,*,#4072,.F.);
#5456=ORIENTED_EDGE('',*,*,#4091,.T.);
#5457=ORIENTED_EDGE('',*,*,#3991,.F.);
#5458=ORIENTED_EDGE('',*,*,#4076,.T.);
#5459=ORIENTED_EDGE('',*,*,#4092,.T.);
#5460=ORIENTED_EDGE('',*,*,#4081,.T.);
#5461=ORIENTED_EDGE('',*,*,#4093,.T.);
#5462=ORIENTED_EDGE('',*,*,#4074,.F.);
#5463=ORIENTED_EDGE('',*,*,#4094,.T.);
#5464=ORIENTED_EDGE('',*,*,#4086,.T.);
#5465=ORIENTED_EDGE('',*,*,#4095,.T.);
#5466=ORIENTED_EDGE('',*,*,#3989,.F.);
#5467=ORIENTED_EDGE('',*,*,#3988,.T.);
#5468=ORIENTED_EDGE('',*,*,#3983,.F.);
#5469=ORIENTED_EDGE('',*,*,#4089,.F.);
#5470=ORIENTED_EDGE('',*,*,#4077,.F.);
#5471=ORIENTED_EDGE('',*,*,#4095,.F.);
#5472=ORIENTED_EDGE('',*,*,#4085,.F.);
#5473=ORIENTED_EDGE('',*,*,#4092,.F.);
#5474=ORIENTED_EDGE('',*,*,#4080,.F.);
#5475=ORIENTED_EDGE('',*,*,#4060,.F.);
#5476=ORIENTED_EDGE('',*,*,#4082,.F.);
#5477=ORIENTED_EDGE('',*,*,#4068,.F.);
#5478=ORIENTED_EDGE('',*,*,#4079,.F.);
#5479=ORIENTED_EDGE('',*,*,#4088,.F.);
#5480=ORIENTED_EDGE('',*,*,#4037,.F.);
#5481=ORIENTED_EDGE('',*,*,#4091,.F.);
#5482=ORIENTED_EDGE('',*,*,#4071,.F.);
#5483=ORIENTED_EDGE('',*,*,#4069,.F.);
#5484=ORIENTED_EDGE('',*,*,#4039,.F.);
#5485=ORIENTED_EDGE('',*,*,#4064,.F.);
#5486=ORIENTED_EDGE('',*,*,#4075,.F.);
#5487=ORIENTED_EDGE('',*,*,#4093,.F.);
#5488=ORIENTED_EDGE('',*,*,#4083,.F.);
#5489=ORIENTED_EDGE('',*,*,#4090,.F.);
#5490=ORIENTED_EDGE('',*,*,#4087,.F.);
#5491=ORIENTED_EDGE('',*,*,#4094,.F.);
#5492=ORIENTED_EDGE('',*,*,#4073,.F.);
#5493=ORIENTED_EDGE('',*,*,#4096,.T.);
#5494=ORIENTED_EDGE('',*,*,#4097,.T.);
#5495=ORIENTED_EDGE('',*,*,#4098,.T.);
#5496=ORIENTED_EDGE('',*,*,#4099,.T.);
#5497=ORIENTED_EDGE('',*,*,#4100,.T.);
#5498=ORIENTED_EDGE('',*,*,#4101,.T.);
#5499=ORIENTED_EDGE('',*,*,#4096,.F.);
#5500=ORIENTED_EDGE('',*,*,#4102,.T.);
#5501=ORIENTED_EDGE('',*,*,#4103,.F.);
#5502=ORIENTED_EDGE('',*,*,#4042,.T.);
#5503=ORIENTED_EDGE('',*,*,#3982,.F.);
#5504=ORIENTED_EDGE('',*,*,#4104,.T.);
#5505=ORIENTED_EDGE('',*,*,#4105,.T.);
#5506=ORIENTED_EDGE('',*,*,#4100,.F.);
#5507=ORIENTED_EDGE('',*,*,#4041,.T.);
#5508=ORIENTED_EDGE('',*,*,#4098,.F.);
#5509=ORIENTED_EDGE('',*,*,#4106,.T.);
#5510=ORIENTED_EDGE('',*,*,#4104,.F.);
#5511=ORIENTED_EDGE('',*,*,#4044,.T.);
#5512=ORIENTED_EDGE('',*,*,#4107,.T.);
#5513=ORIENTED_EDGE('',*,*,#4108,.T.);
#5514=ORIENTED_EDGE('',*,*,#3980,.F.);
#5515=ORIENTED_EDGE('',*,*,#4103,.T.);
#5516=ORIENTED_EDGE('',*,*,#4109,.T.);
#5517=ORIENTED_EDGE('',*,*,#4107,.F.);
#5518=ORIENTED_EDGE('',*,*,#4043,.T.);
#5519=ORIENTED_EDGE('',*,*,#4101,.F.);
#5520=ORIENTED_EDGE('',*,*,#4105,.F.);
#5521=ORIENTED_EDGE('',*,*,#4106,.F.);
#5522=ORIENTED_EDGE('',*,*,#4097,.F.);
#5523=ORIENTED_EDGE('',*,*,#4108,.F.);
#5524=ORIENTED_EDGE('',*,*,#4109,.F.);
#5525=ORIENTED_EDGE('',*,*,#4102,.F.);
#5526=ORIENTED_EDGE('',*,*,#4099,.F.);
#5527=ORIENTED_EDGE('',*,*,#4050,.F.);
#5528=ORIENTED_EDGE('',*,*,#4025,.F.);
#5529=ORIENTED_EDGE('',*,*,#4015,.F.);
#5530=ORIENTED_EDGE('',*,*,#4031,.F.);
#5531=ORIENTED_EDGE('',*,*,#4005,.F.);
#5532=ORIENTED_EDGE('',*,*,#4022,.F.);
#5533=ORIENTED_EDGE('',*,*,#4055,.F.);
#5534=ORIENTED_EDGE('',*,*,#4033,.F.);
#5535=ORIENTED_EDGE('',*,*,#4029,.F.);
#5536=ORIENTED_EDGE('',*,*,#4018,.T.);
#5537=ORIENTED_EDGE('',*,*,#4110,.T.);
#5538=ORIENTED_EDGE('',*,*,#4048,.F.);
#5539=ORIENTED_EDGE('',*,*,#4053,.F.);
#5540=ORIENTED_EDGE('',*,*,#4111,.T.);
#5541=ORIENTED_EDGE('',*,*,#4002,.T.);
#5542=ORIENTED_EDGE('',*,*,#4049,.F.);
#5543=ORIENTED_EDGE('',*,*,#4110,.F.);
#5544=ORIENTED_EDGE('',*,*,#4017,.F.);
#5545=ORIENTED_EDGE('',*,*,#4024,.F.);
#5546=ORIENTED_EDGE('',*,*,#4003,.F.);
#5547=ORIENTED_EDGE('',*,*,#4111,.F.);
#5548=ORIENTED_EDGE('',*,*,#4052,.F.);
#5549=ORIENTED_EDGE('',*,*,#4020,.F.);
#6451=TOROIDAL_SURFACE('',#7384,8.16998586739121,2.);
#6600=ADVANCED_FACE('',(#1948),#1705,.F.);
#6601=ADVANCED_FACE('',(#1949),#1706,.T.);
#6602=ADVANCED_FACE('',(#1950),#1707,.T.);
#6603=ADVANCED_FACE('',(#1951),#1708,.T.);
#6604=ADVANCED_FACE('',(#1952),#1709,.F.);
#6605=ADVANCED_FACE('',(#1953),#1710,.F.);
#6606=ADVANCED_FACE('',(#1954,#312,#313),#121,.T.);
#6607=ADVANCED_FACE('',(#1955),#1711,.F.);
#6608=ADVANCED_FACE('',(#1956),#1712,.F.);
#6609=ADVANCED_FACE('',(#1957,#314),#6451,.T.);
#6610=ADVANCED_FACE('',(#1958),#1713,.F.);
#6611=ADVANCED_FACE('',(#1959),#463,.T.);
#6612=ADVANCED_FACE('',(#1960),#122,.T.);
#6613=ADVANCED_FACE('',(#1961,#315),#1714,.T.);
#6614=ADVANCED_FACE('',(#1962),#464,.T.);
#6615=ADVANCED_FACE('',(#1963,#316),#465,.T.);
#6616=ADVANCED_FACE('',(#1964,#317),#466,.T.);
#6617=ADVANCED_FACE('',(#1965),#467,.F.);
#6618=ADVANCED_FACE('',(#1966),#468,.F.);
#6619=ADVANCED_FACE('',(#1967,#318),#469,.F.);
#6620=ADVANCED_FACE('',(#1968),#470,.F.);
#6621=ADVANCED_FACE('',(#1969,#319),#471,.F.);
#6622=ADVANCED_FACE('',(#1970),#472,.F.);
#6623=ADVANCED_FACE('',(#1971),#473,.F.);
#6624=ADVANCED_FACE('',(#1972),#474,.T.);
#6625=ADVANCED_FACE('',(#1973),#475,.F.);
#6626=ADVANCED_FACE('',(#1974,#320),#476,.F.);
#6627=ADVANCED_FACE('',(#1975,#321),#477,.F.);
#6628=ADVANCED_FACE('',(#1976),#478,.T.);
#6629=ADVANCED_FACE('',(#1977),#479,.F.);
#6630=ADVANCED_FACE('',(#1978),#1715,.T.);
#6631=ADVANCED_FACE('',(#1979),#1716,.T.);
#6632=ADVANCED_FACE('',(#1980),#1717,.T.);
#6633=ADVANCED_FACE('',(#1981),#1718,.T.);
#6634=ADVANCED_FACE('',(#1982),#1719,.T.);
#6635=ADVANCED_FACE('',(#1983),#1720,.T.);
#6636=ADVANCED_FACE('',(#1984),#480,.F.);
#6637=ADVANCED_FACE('',(#1985,#322),#481,.T.);
#6638=ADVANCED_FACE('',(#1986),#482,.T.);
#6639=ADVANCED_FACE('',(#1987,#323),#483,.T.);
#6640=ADVANCED_FACE('',(#1988),#484,.T.);
#6641=ADVANCED_FACE('',(#1989),#1721,.T.);
#6642=ADVANCED_FACE('',(#1990),#1722,.T.);
#6643=ADVANCED_FACE('',(#1991),#1723,.T.);
#6644=ADVANCED_FACE('',(#1992),#1724,.T.);
#6645=ADVANCED_FACE('',(#1993),#1725,.F.);
#6646=ADVANCED_FACE('',(#1994),#1726,.F.);
#6647=ADVANCED_FACE('',(#1995),#1727,.F.);
#6648=ADVANCED_FACE('',(#1996),#1728,.T.);
#6649=ADVANCED_FACE('',(#1997),#1729,.T.);
#6846=CLOSED_SHELL('',(#6600,#6601,#6602,#6603,#6604,#6605,#6606,#6607,
#6608,#6609,#6610,#6611,#6612,#6613,#6614,#6615,#6616,#6617,#6618,#6619,
#6620,#6621,#6622,#6623,#6624,#6625,#6626,#6627,#6628,#6629,#6630,#6631,
#6632,#6633,#6634,#6635,#6636,#6637,#6638,#6639,#6640,#6641,#6642,#6643,
#6644,#6645,#6646,#6647,#6648,#6649));
#7359=AXIS2_PLACEMENT_3D('',#11047,#8612,#8613);
#7360=AXIS2_PLACEMENT_3D('',#11048,#8614,#8615);
#7361=AXIS2_PLACEMENT_3D('',#11050,#8616,#8617);
#7362=AXIS2_PLACEMENT_3D('',#11053,#8619,#8620);
#7363=AXIS2_PLACEMENT_3D('',#11054,#8621,#8622);
#7364=AXIS2_PLACEMENT_3D('',#11056,#8623,#8624);
#7365=AXIS2_PLACEMENT_3D('',#11059,#8626,#8627);
#7366=AXIS2_PLACEMENT_3D('',#11060,#8628,#8629);
#7367=AXIS2_PLACEMENT_3D('',#11062,#8630,#8631);
#7368=AXIS2_PLACEMENT_3D('',#11065,#8633,#8634);
#7369=AXIS2_PLACEMENT_3D('',#11066,#8635,#8636);
#7370=AXIS2_PLACEMENT_3D('',#11068,#8637,#8638);
#7371=AXIS2_PLACEMENT_3D('',#11071,#8640,#8641);
#7372=AXIS2_PLACEMENT_3D('',#11072,#8642,#8643);
#7373=AXIS2_PLACEMENT_3D('',#11074,#8644,#8645);
#7374=AXIS2_PLACEMENT_3D('',#11115,#8647,#8648);
#7375=AXIS2_PLACEMENT_3D('',#11138,#8650,#8651);
#7376=AXIS2_PLACEMENT_3D('',#11158,#8652,#8653);
#7377=AXIS2_PLACEMENT_3D('',#11161,#8654,#8655);
#7378=AXIS2_PLACEMENT_3D('',#11219,#8656,#8657);
#7379=AXIS2_PLACEMENT_3D('',#11260,#8659,#8660);
#7380=AXIS2_PLACEMENT_3D('',#11316,#8661,#8662);
#7381=AXIS2_PLACEMENT_3D('',#11320,#8664,#8665);
#7382=AXIS2_PLACEMENT_3D('',#11322,#8667,#8668);
#7383=AXIS2_PLACEMENT_3D('',#11325,#8669,#8670);
#7384=AXIS2_PLACEMENT_3D('',#11328,#8673,#8674);
#7385=AXIS2_PLACEMENT_3D('',#11331,#8675,#8676);
#7386=AXIS2_PLACEMENT_3D('',#11411,#8677,#8678);
#7387=AXIS2_PLACEMENT_3D('',#11414,#8679,#8680);
#7388=AXIS2_PLACEMENT_3D('',#11425,#8683,#8684);
#7389=AXIS2_PLACEMENT_3D('',#11427,#8686,#8687);
#7390=AXIS2_PLACEMENT_3D('',#11436,#8692,#8693);
#7391=AXIS2_PLACEMENT_3D('',#11437,#8694,#8695);
#7392=AXIS2_PLACEMENT_3D('',#11438,#8696,#8697);
#7393=AXIS2_PLACEMENT_3D('',#11443,#8699,#8700);
#7394=AXIS2_PLACEMENT_3D('',#11446,#8702,#8703);
#7395=AXIS2_PLACEMENT_3D('',#11447,#8704,#8705);
#7396=AXIS2_PLACEMENT_3D('',#11453,#8709,#8710);
#7397=AXIS2_PLACEMENT_3D('',#11455,#8711,#8712);
#7398=AXIS2_PLACEMENT_3D('',#11456,#8713,#8714);
#7399=AXIS2_PLACEMENT_3D('',#11457,#8715,#8716);
#7400=AXIS2_PLACEMENT_3D('',#11459,#8718,#8719);
#7401=AXIS2_PLACEMENT_3D('',#11461,#8720,#8721);
#7402=AXIS2_PLACEMENT_3D('',#11462,#8722,#8723);
#7403=AXIS2_PLACEMENT_3D('',#11464,#8725,#8726);
#7404=AXIS2_PLACEMENT_3D('',#11465,#8727,#8728);
#7405=AXIS2_PLACEMENT_3D('',#11466,#8729,#8730);
#7406=AXIS2_PLACEMENT_3D('',#11472,#8734,#8735);
#7407=AXIS2_PLACEMENT_3D('',#11477,#8737,#8738);
#7408=AXIS2_PLACEMENT_3D('',#11483,#8742,#8743);
#7409=AXIS2_PLACEMENT_3D('',#11484,#8744,#8745);
#7410=AXIS2_PLACEMENT_3D('',#11488,#8748,#8749);
#7411=AXIS2_PLACEMENT_3D('',#11491,#8751,#8752);
#7412=AXIS2_PLACEMENT_3D('',#11493,#8753,#8754);
#7413=AXIS2_PLACEMENT_3D('',#11495,#8756,#8757);
#7414=AXIS2_PLACEMENT_3D('',#11505,#8763,#8764);
#7415=AXIS2_PLACEMENT_3D('',#11515,#8770,#8771);
#7416=AXIS2_PLACEMENT_3D('',#11521,#8775,#8776);
#7417=AXIS2_PLACEMENT_3D('',#11530,#8781,#8782);
#7418=AXIS2_PLACEMENT_3D('',#11531,#8783,#8784);
#7419=AXIS2_PLACEMENT_3D('',#11532,#8785,#8786);
#7420=AXIS2_PLACEMENT_3D('',#11533,#8787,#8788);
#7421=AXIS2_PLACEMENT_3D('',#11534,#8789,#8790);
#7422=AXIS2_PLACEMENT_3D('',#11535,#8791,#8792);
#7423=AXIS2_PLACEMENT_3D('',#11536,#8793,#8794);
#7424=AXIS2_PLACEMENT_3D('',#11537,#8795,#8796);
#7425=AXIS2_PLACEMENT_3D('',#11538,#8797,#8798);
#7426=AXIS2_PLACEMENT_3D('',#11539,#8799,#8800);
#7427=AXIS2_PLACEMENT_3D('',#11540,#8801,#8802);
#7428=AXIS2_PLACEMENT_3D('',#11541,#8803,#8804);
#7429=AXIS2_PLACEMENT_3D('',#11542,#8805,#8806);
#7430=AXIS2_PLACEMENT_3D('',#11543,#8807,#8808);
#7431=AXIS2_PLACEMENT_3D('',#11544,#8809,#8810);
#7432=AXIS2_PLACEMENT_3D('',#11545,#8811,#8812);
#7433=AXIS2_PLACEMENT_3D('',#11546,#8813,#8814);
#7434=AXIS2_PLACEMENT_3D('',#11547,#8815,#8816);
#7435=AXIS2_PLACEMENT_3D('',#11548,#8817,#8818);
#7436=AXIS2_PLACEMENT_3D('',#11557,#8823,#8824);
#7437=AXIS2_PLACEMENT_3D('',#11560,#8826,#8827);
#7438=AXIS2_PLACEMENT_3D('',#11562,#8828,#8829);
#7439=AXIS2_PLACEMENT_3D('',#11564,#8831,#8832);
#7440=AXIS2_PLACEMENT_3D('',#11568,#8835,#8836);
#7441=AXIS2_PLACEMENT_3D('',#11569,#8837,#8838);
#7442=AXIS2_PLACEMENT_3D('',#11572,#8840,#8841);
#7443=AXIS2_PLACEMENT_3D('',#11573,#8842,#8843);
#7444=AXIS2_PLACEMENT_3D('',#11575,#8845,#8846);
#7445=AXIS2_PLACEMENT_3D('',#11576,#8847,#8848);
#7446=AXIS2_PLACEMENT_3D('',#11577,#8849,#8850);
#7447=AXIS2_PLACEMENT_3D('',#11578,#8851,#8852);
#7448=AXIS2_PLACEMENT_3D('',#11579,#8853,#8854);
#7449=AXIS2_PLACEMENT_3D('',#11580,#8855,#8856);
#7450=AXIS2_PLACEMENT_3D('',#11582,#8858,#8859);
#7451=AXIS2_PLACEMENT_3D('',#11584,#8861,#8862);
#7452=AXIS2_PLACEMENT_3D('',#11585,#8863,#8864);
#8612=DIRECTION('axis',(0.,0.,1.));
#8613=DIRECTION('refdir',(1.,0.,0.));
#8614=DIRECTION('center_axis',(0.,-1.,0.));
#8615=DIRECTION('ref_axis',(0.,0.,-1.));
#8616=DIRECTION('center_axis',(0.,1.,0.));
#8617=DIRECTION('ref_axis',(0.,0.,1.));
#8618=DIRECTION('',(0.,-1.,0.));
#8619=DIRECTION('center_axis',(0.,-1.,0.));
#8620=DIRECTION('ref_axis',(0.,0.,-1.));
#8621=DIRECTION('center_axis',(0.,1.,0.));
#8622=DIRECTION('ref_axis',(0.,0.,1.));
#8623=DIRECTION('center_axis',(0.,-1.,0.));
#8624=DIRECTION('ref_axis',(0.,0.,-1.));
#8625=DIRECTION('',(0.,-1.,0.));
#8626=DIRECTION('center_axis',(0.,1.,0.));
#8627=DIRECTION('ref_axis',(0.,0.,-1.));
#8628=DIRECTION('center_axis',(0.,1.,0.));
#8629=DIRECTION('ref_axis',(0.,0.,1.));
#8630=DIRECTION('center_axis',(0.,-1.,0.));
#8631=DIRECTION('ref_axis',(0.,0.,1.));
#8632=DIRECTION('',(0.,-1.,0.));
#8633=DIRECTION('center_axis',(0.,-1.,0.));
#8634=DIRECTION('ref_axis',(0.,0.,-1.));
#8635=DIRECTION('center_axis',(0.,1.,0.));
#8636=DIRECTION('ref_axis',(0.,0.,1.));
#8637=DIRECTION('center_axis',(0.,-1.,0.));
#8638=DIRECTION('ref_axis',(0.,0.,1.));
#8639=DIRECTION('',(0.,-1.,0.));
#8640=DIRECTION('center_axis',(0.,1.,0.));
#8641=DIRECTION('ref_axis',(0.,0.,-1.));
#8642=DIRECTION('center_axis',(0.,-1.,0.));
#8643=DIRECTION('ref_axis',(0.,0.,-1.));
#8644=DIRECTION('center_axis',(0.,-1.,-1.24352412568707E-16));
#8645=DIRECTION('ref_axis',(0.,-1.24352412568707E-16,1.));
#8646=DIRECTION('',(0.,-1.,0.));
#8647=DIRECTION('center_axis',(0.,-1.,0.));
#8648=DIRECTION('ref_axis',(0.,0.,-1.));
#8649=DIRECTION('',(0.,-1.,0.));
#8650=DIRECTION('center_axis',(0.,1.,1.24352412568707E-16));
#8651=DIRECTION('ref_axis',(0.,1.24352412568707E-16,-1.));
#8652=DIRECTION('center_axis',(0.,0.,-1.));
#8653=DIRECTION('ref_axis',(1.,0.,0.));
#8654=DIRECTION('center_axis',(0.,0.,1.));
#8655=DIRECTION('ref_axis',(-1.,0.,0.));
#8656=DIRECTION('center_axis',(0.,0.,1.));
#8657=DIRECTION('ref_axis',(-1.,0.,0.));
#8658=DIRECTION('',(0.0174524064372835,-2.1373033680838E-18,0.999847695156391));
#8659=DIRECTION('center_axis',(0.,0.,1.));
#8660=DIRECTION('ref_axis',(-1.,0.,0.));
#8661=DIRECTION('center_axis',(0.,-1.,0.));
#8662=DIRECTION('ref_axis',(0.,0.,-1.));
#8663=DIRECTION('',(0.,-1.,0.));
#8664=DIRECTION('center_axis',(0.,1.,1.24352412568707E-16));
#8665=DIRECTION('ref_axis',(0.,1.24352412568707E-16,-1.));
#8666=DIRECTION('',(0.,1.,0.));
#8667=DIRECTION('center_axis',(0.,-1.,0.));
#8668=DIRECTION('ref_axis',(0.,0.,-1.));
#8669=DIRECTION('center_axis',(0.,-1.,-1.24352412568707E-16));
#8670=DIRECTION('ref_axis',(1.86381695289753E-15,-1.24352412568707E-16,
1.));
#8671=DIRECTION('',(0.,-1.,0.));
#8672=DIRECTION('',(0.,1.,0.));
#8673=DIRECTION('center_axis',(0.,1.15648231731787E-16,-1.));
#8674=DIRECTION('ref_axis',(0.,1.,0.));
#8675=DIRECTION('center_axis',(0.,1.15648231731787E-16,-1.));
#8676=DIRECTION('ref_axis',(0.,1.,1.15648231731787E-16));
#8677=DIRECTION('center_axis',(0.,-1.,0.));
#8678=DIRECTION('ref_axis',(0.,0.,-1.));
#8679=DIRECTION('center_axis',(0.,1.,1.24352412568707E-16));
#8680=DIRECTION('ref_axis',(0.,-1.24352412568707E-16,1.));
#8681=DIRECTION('',(0.,-1.,0.));
#8682=DIRECTION('',(0.,-1.,0.));
#8683=DIRECTION('center_axis',(0.,-1.,-1.24352412568707E-16));
#8684=DIRECTION('ref_axis',(0.,1.24352412568707E-16,-1.));
#8685=DIRECTION('',(0.,1.,0.));
#8686=DIRECTION('center_axis',(-0.707106781186547,0.,-0.707106781186548));
#8687=DIRECTION('ref_axis',(-0.707106781186548,0.,0.707106781186547));
#8688=DIRECTION('',(-0.707106781186548,0.,0.707106781186547));
#8689=DIRECTION('',(0.,1.,0.));
#8690=DIRECTION('',(-0.707106781186548,0.,0.707106781186547));
#8691=DIRECTION('',(0.,-1.,0.));
#8692=DIRECTION('center_axis',(0.,0.,-1.));
#8693=DIRECTION('ref_axis',(-1.,-1.22464679914735E-16,0.));
#8694=DIRECTION('center_axis',(0.,0.,-1.));
#8695=DIRECTION('ref_axis',(1.,1.77635684317072E-15,0.));
#8696=DIRECTION('center_axis',(0.,-1.,0.));
#8697=DIRECTION('ref_axis',(3.0760962761356E-5,0.,0.999999999526882));
#8698=DIRECTION('',(0.,1.,0.));
#8699=DIRECTION('center_axis',(0.,1.,0.));
#8700=DIRECTION('ref_axis',(2.66489596482314E-15,0.,-1.));
#8701=DIRECTION('',(0.,-1.,0.));
#8702=DIRECTION('center_axis',(0.,-1.,0.));
#8703=DIRECTION('ref_axis',(0.,0.,1.));
#8704=DIRECTION('center_axis',(0.,1.15648231731787E-16,-1.));
#8705=DIRECTION('ref_axis',(0.,1.,1.15648231731787E-16));
#8706=DIRECTION('',(-1.,0.,0.));
#8707=DIRECTION('',(0.,-1.,-1.15648231731787E-16));
#8708=DIRECTION('',(-1.,0.,0.));
#8709=DIRECTION('center_axis',(0.,1.,1.24352412568707E-16));
#8710=DIRECTION('ref_axis',(0.,-1.24352412568707E-16,1.));
#8711=DIRECTION('center_axis',(0.,-1.,-1.24352412568707E-16));
#8712=DIRECTION('ref_axis',(0.,-1.24352412568707E-16,1.));
#8713=DIRECTION('center_axis',(0.,1.,1.24352412568707E-16));
#8714=DIRECTION('ref_axis',(0.,-1.24352412568707E-16,1.));
#8715=DIRECTION('center_axis',(0.,1.,1.24352412568707E-16));
#8716=DIRECTION('ref_axis',(0.,-1.24352412568707E-16,1.));
#8717=DIRECTION('',(0.,1.24352412568707E-16,-1.));
#8718=DIRECTION('center_axis',(0.,-1.,-1.24352412568707E-16));
#8719=DIRECTION('ref_axis',(0.,1.24352412568707E-16,-1.));
#8720=DIRECTION('center_axis',(0.,-1.,-1.24352412568707E-16));
#8721=DIRECTION('ref_axis',(0.,1.24352412568707E-16,-1.));
#8722=DIRECTION('center_axis',(0.,1.,1.24352412568707E-16));
#8723=DIRECTION('ref_axis',(0.,1.24352412568707E-16,-1.));
#8724=DIRECTION('',(0.,-1.24352412568707E-16,1.));
#8725=DIRECTION('center_axis',(0.,-1.,-1.24352412568707E-16));
#8726=DIRECTION('ref_axis',(0.,1.24352412568707E-16,-1.));
#8727=DIRECTION('center_axis',(-1.,0.,0.));
#8728=DIRECTION('ref_axis',(0.,0.,1.));
#8729=DIRECTION('center_axis',(0.,0.,1.));
#8730=DIRECTION('ref_axis',(1.,0.,0.));
#8731=DIRECTION('',(-1.,0.,0.));
#8732=DIRECTION('',(0.,1.,0.));
#8733=DIRECTION('',(-1.,0.,0.));
#8734=DIRECTION('center_axis',(0.,-1.,0.));
#8735=DIRECTION('ref_axis',(0.,0.,-1.));
#8736=DIRECTION('',(0.707106781186548,0.,-0.707106781186547));
#8737=DIRECTION('center_axis',(0.,1.,0.));
#8738=DIRECTION('ref_axis',(0.,0.,-1.));
#8739=DIRECTION('',(0.707106781186548,0.,0.707106781186548));
#8740=DIRECTION('',(-1.,0.,0.));
#8741=DIRECTION('',(0.707106781186548,0.,0.707106781186548));
#8742=DIRECTION('center_axis',(0.,1.,0.));
#8743=DIRECTION('ref_axis',(-4.33680868994202E-15,0.,-1.));
#8744=DIRECTION('center_axis',(0.,0.,-1.));
#8745=DIRECTION('ref_axis',(-1.,0.,0.));
#8746=DIRECTION('',(0.,-1.,0.));
#8747=DIRECTION('',(-1.,0.,0.));
#8748=DIRECTION('center_axis',(0.,1.,0.));
#8749=DIRECTION('ref_axis',(0.,0.,1.));
#8750=DIRECTION('',(0.707106781186548,0.,0.707106781186548));
#8751=DIRECTION('center_axis',(0.,-1.,0.));
#8752=DIRECTION('ref_axis',(0.,0.,1.));
#8753=DIRECTION('center_axis',(0.,-1.,0.));
#8754=DIRECTION('ref_axis',(-2.16840434497101E-15,0.,1.));
#8755=DIRECTION('',(0.707106781186548,0.,0.707106781186548));
#8756=DIRECTION('center_axis',(-0.707106781186548,0.,0.707106781186547));
#8757=DIRECTION('ref_axis',(0.707106781186547,0.,0.707106781186548));
#8758=DIRECTION('',(0.,1.,0.));
#8759=DIRECTION('',(0.707106781186548,0.,0.707106781186548));
#8760=DIRECTION('',(0.,1.,0.));
#8761=DIRECTION('',(-0.707106781186548,0.,-0.707106781186548));
#8762=DIRECTION('',(0.,1.,0.));
#8763=DIRECTION('center_axis',(0.707106781186548,0.,-0.707106781186547));
#8764=DIRECTION('ref_axis',(-0.707106781186547,0.,-0.707106781186548));
#8765=DIRECTION('',(-0.707106781186548,0.,-0.707106781186548));
#8766=DIRECTION('',(0.,-1.,0.));
#8767=DIRECTION('',(0.707106781186548,0.,0.707106781186548));
#8768=DIRECTION('',(0.,-1.,0.));
#8769=DIRECTION('',(0.,-1.,0.));
#8770=DIRECTION('center_axis',(-0.707106781186547,0.,-0.707106781186548));
#8771=DIRECTION('ref_axis',(-0.707106781186548,0.,0.707106781186547));
#8772=DIRECTION('',(0.707106781186548,0.,-0.707106781186547));
#8773=DIRECTION('',(0.,1.,0.));
#8774=DIRECTION('',(0.,-1.,0.));
#8775=DIRECTION('center_axis',(0.707106781186548,0.,0.707106781186548));
#8776=DIRECTION('ref_axis',(0.707106781186548,0.,-0.707106781186548));
#8777=DIRECTION('',(-0.707106781186547,0.,0.707106781186547));
#8778=DIRECTION('',(0.,1.,0.));
#8779=DIRECTION('',(-0.707106781186547,0.,0.707106781186547));
#8780=DIRECTION('',(0.,-1.,0.));
#8781=DIRECTION('center_axis',(0.,-1.,0.));
#8782=DIRECTION('ref_axis',(0.,0.,-1.));
#8783=DIRECTION('center_axis',(0.,1.,0.));
#8784=DIRECTION('ref_axis',(-4.33680868994202E-15,0.,-1.));
#8785=DIRECTION('center_axis',(0.,-1.,0.));
#8786=DIRECTION('ref_axis',(0.,0.,-1.));
#8787=DIRECTION('center_axis',(0.,-1.,0.));
#8788=DIRECTION('ref_axis',(0.,0.,-1.));
#8789=DIRECTION('center_axis',(0.,1.,0.));
#8790=DIRECTION('ref_axis',(-4.33680868994202E-15,0.,-1.));
#8791=DIRECTION('center_axis',(0.,1.,0.));
#8792=DIRECTION('ref_axis',(0.,0.,1.));
#8793=DIRECTION('center_axis',(0.,-1.,0.));
#8794=DIRECTION('ref_axis',(0.,0.,1.));
#8795=DIRECTION('center_axis',(0.,-1.,0.));
#8796=DIRECTION('ref_axis',(-2.16840434497101E-15,0.,1.));
#8797=DIRECTION('center_axis',(0.,1.,0.));
#8798=DIRECTION('ref_axis',(0.,0.,1.));
#8799=DIRECTION('center_axis',(0.,1.,0.));
#8800=DIRECTION('ref_axis',(0.,0.,1.));
#8801=DIRECTION('center_axis',(0.,-1.,0.));
#8802=DIRECTION('ref_axis',(0.,0.,-1.));
#8803=DIRECTION('center_axis',(0.,-1.,0.));
#8804=DIRECTION('ref_axis',(0.,0.,-1.));
#8805=DIRECTION('center_axis',(0.,1.,0.));
#8806=DIRECTION('ref_axis',(0.,0.,1.));
#8807=DIRECTION('center_axis',(0.,-1.,0.));
#8808=DIRECTION('ref_axis',(0.,0.,-1.));
#8809=DIRECTION('center_axis',(0.,-1.,0.));
#8810=DIRECTION('ref_axis',(0.,0.,-1.));
#8811=DIRECTION('center_axis',(0.,1.,0.));
#8812=DIRECTION('ref_axis',(1.45473230946492E-15,0.,-1.));
#8813=DIRECTION('center_axis',(0.,1.,0.));
#8814=DIRECTION('ref_axis',(1.45473230946492E-15,0.,-1.));
#8815=DIRECTION('center_axis',(0.,1.,0.));
#8816=DIRECTION('ref_axis',(1.01064309961486E-15,0.,-1.));
#8817=DIRECTION('center_axis',(0.,0.,-1.));
#8818=DIRECTION('ref_axis',(-1.,0.,0.));
#8819=DIRECTION('',(1.,0.,0.));
#8820=DIRECTION('',(0.,1.,0.));
#8821=DIRECTION('',(-1.,0.,0.));
#8822=DIRECTION('',(0.,-1.,0.));
#8823=DIRECTION('center_axis',(0.,-1.,0.));
#8824=DIRECTION('ref_axis',(0.,0.,-1.));
#8825=DIRECTION('',(0.,0.,1.));
#8826=DIRECTION('center_axis',(0.,-1.,0.));
#8827=DIRECTION('ref_axis',(0.,0.,-1.));
#8828=DIRECTION('center_axis',(0.,-1.,0.));
#8829=DIRECTION('ref_axis',(0.,0.,-1.));
#8830=DIRECTION('',(0.,0.,1.));
#8831=DIRECTION('center_axis',(1.,0.,0.));
#8832=DIRECTION('ref_axis',(0.,0.,-1.));
#8833=DIRECTION('',(0.,0.,1.));
#8834=DIRECTION('',(0.,-1.,0.));
#8835=DIRECTION('center_axis',(0.,1.,0.));
#8836=DIRECTION('ref_axis',(0.,0.,1.));
#8837=DIRECTION('center_axis',(0.,1.,0.));
#8838=DIRECTION('ref_axis',(0.,0.,1.));
#8839=DIRECTION('',(0.,0.,1.));
#8840=DIRECTION('center_axis',(0.,1.,0.));
#8841=DIRECTION('ref_axis',(0.,0.,1.));
#8842=DIRECTION('center_axis',(-1.,0.,0.));
#8843=DIRECTION('ref_axis',(0.,0.,1.));
#8844=DIRECTION('',(0.,1.,0.));
#8845=DIRECTION('center_axis',(0.,-1.,0.));
#8846=DIRECTION('ref_axis',(0.,0.,-1.));
#8847=DIRECTION('center_axis',(0.,1.,0.));
#8848=DIRECTION('ref_axis',(0.,0.,1.));
#8849=DIRECTION('center_axis',(0.,-1.,0.));
#8850=DIRECTION('ref_axis',(0.,0.,-1.));
#8851=DIRECTION('center_axis',(0.,-1.,0.));
#8852=DIRECTION('ref_axis',(0.,0.,-1.));
#8853=DIRECTION('center_axis',(0.,-1.,0.));
#8854=DIRECTION('ref_axis',(0.,0.,-1.));
#8855=DIRECTION('center_axis',(0.,-1.,0.));
#8856=DIRECTION('ref_axis',(0.,0.,-1.));
#8857=DIRECTION('',(0.,1.,0.));
#8858=DIRECTION('center_axis',(0.,-1.,0.));
#8859=DIRECTION('ref_axis',(0.,0.,-1.));
#8860=DIRECTION('',(0.,1.,0.));
#8861=DIRECTION('center_axis',(0.,-1.,0.));
#8862=DIRECTION('ref_axis',(0.,0.,-1.));
#8863=DIRECTION('center_axis',(0.,-1.,0.));
#8864=DIRECTION('ref_axis',(0.,0.,-1.));
#11047=CARTESIAN_POINT('',(0.,0.,0.));
#11048=CARTESIAN_POINT('Origin',(-0.178867612462208,4.46390384366945,37.06975632091));
#11049=CARTESIAN_POINT('',(-0.178867612462208,3.53610097918737,38.26975632091));
#11050=CARTESIAN_POINT('Origin',(-0.178867612462208,3.53610097918737,37.06975632091));
#11051=CARTESIAN_POINT('',(-0.178867612462208,-3.53609615633055,38.26975632091));
#11052=CARTESIAN_POINT('',(-0.178867612462208,4.46390384366945,38.26975632091));
#11053=CARTESIAN_POINT('Origin',(-0.178867612462208,-3.53609615633055,37.06975632091));
#11054=CARTESIAN_POINT('Origin',(-14.6061395505208,-4.33609615633055,3.29091815733825));
#11055=CARTESIAN_POINT('',(-14.6061395505208,4.33590384366945,2.49091815733825));
#11056=CARTESIAN_POINT('Origin',(-14.6061395505208,4.33590384366945,3.29091815733825));
#11057=CARTESIAN_POINT('',(-14.6061395505208,3.53610097918737,2.49091815733825));
#11058=CARTESIAN_POINT('',(-14.6061395505208,-4.33609615633055,2.49091815733825));
#11059=CARTESIAN_POINT('Origin',(-14.6061395505208,3.53610097918737,3.29091815733825));
#11060=CARTESIAN_POINT('Origin',(-14.6061395505208,-4.33609615633055,3.29091815733825));
#11061=CARTESIAN_POINT('',(-14.6061395505208,-3.53609615633055,2.49091815733825));
#11062=CARTESIAN_POINT('Origin',(-14.6061395505208,-3.53609615633055,3.29091815733825));
#11063=CARTESIAN_POINT('',(-14.6061395505208,-4.33609615633055,2.49091815733825));
#11064=CARTESIAN_POINT('',(-14.6061395505208,-4.33609615633055,2.49091815733825));
#11065=CARTESIAN_POINT('Origin',(-14.6061395505208,-4.33609615633055,3.29091815733825));
#11066=CARTESIAN_POINT('Origin',(-14.6061395505208,-4.33609615633055,3.29091815733825));
#11067=CARTESIAN_POINT('',(-14.6061395505208,2.00000241142841,2.49091815733825));
#11068=CARTESIAN_POINT('Origin',(-14.6061395505208,2.00000241142841,3.29091815733825));
#11069=CARTESIAN_POINT('',(-14.6061395505208,-1.99999758857159,2.49091815733825));
#11070=CARTESIAN_POINT('',(-14.6061395505208,-4.33609615633055,2.49091815733825));
#11071=CARTESIAN_POINT('Origin',(-14.6061395505208,-1.99999758857159,3.29091815733825));
#11072=CARTESIAN_POINT('Origin',(-0.177712466787677,14.4000024114284,11.6951080862604));
#11073=CARTESIAN_POINT('',(-0.177712466787678,-5.9999975885716,12.8951080862604));
#11074=CARTESIAN_POINT('Origin',(-0.177712466787677,-5.9999975885716,11.6951080862604));
#11075=CARTESIAN_POINT('',(-0.177712466787678,-10.2544850951109,12.8951080862604));
#11076=CARTESIAN_POINT('',(-0.177712466787678,14.4000024114284,12.8951080862604));
#11077=CARTESIAN_POINT('',(-0.177712466787677,-10.2963772509386,10.4951080862604));
#11078=CARTESIAN_POINT('Ctrl Pts',(-0.177712466787677,-10.2544850951109,
12.8951080862604));
#11079=CARTESIAN_POINT('Ctrl Pts',(-0.328316799600617,-10.2544850951109,
12.8951080862604));
#11080=CARTESIAN_POINT('Ctrl Pts',(-0.488902932607147,-10.2513527873625,
12.8650249475386));
#11081=CARTESIAN_POINT('Ctrl Pts',(-0.78426488938881,-10.2402603738984,
12.742790826072));
#11082=CARTESIAN_POINT('Ctrl Pts',(-0.919050045771719,-10.2324873030817,
12.6506454931746));
#11083=CARTESIAN_POINT('Ctrl Pts',(-1.13193181191228,-10.2185593746734,
12.4381249833728));
#11084=CARTESIAN_POINT('Ctrl Pts',(-1.22429085128089,-10.2115028582253,
12.3035493595844));
#11085=CARTESIAN_POINT('Ctrl Pts',(-1.34702914180779,-10.2033604971208,
12.0085177147771));
#11086=CARTESIAN_POINT('Ctrl Pts',(-1.37740318454924,-10.2024688739752,
11.8480541988248));
#11087=CARTESIAN_POINT('Ctrl Pts',(-1.37801799011132,-10.2076973349447,
11.5464521222423));
#11088=CARTESIAN_POINT('Ctrl Pts',(-1.34806997449904,-10.2141906775384,
11.3853937554379));
#11089=CARTESIAN_POINT('Ctrl Pts',(-1.22585140243605,-10.232651025804,11.0892496287149));
#11090=CARTESIAN_POINT('Ctrl Pts',(-1.13359030470793,-10.244422653795,10.9541478187001));
#11091=CARTESIAN_POINT('Ctrl Pts',(-0.920648927729036,-10.2657970316571,
10.7407719255541));
#11092=CARTESIAN_POINT('Ctrl Pts',(-0.785732755478035,-10.2767999672427,
10.6482195366313));
#11093=CARTESIAN_POINT('Ctrl Pts',(-0.489813246463523,-10.2921837256933,
10.5253827273461));
#11094=CARTESIAN_POINT('Ctrl Pts',(-0.328796143270408,-10.2963772509386,
10.4951080862604));
#11095=CARTESIAN_POINT('Ctrl Pts',(-0.177712466787678,-10.2963772509386,
10.4951080862604));
#11096=CARTESIAN_POINT('Ctrl Pts',(-0.177712466787677,-10.2963772509386,
10.4951080862604));
#11097=CARTESIAN_POINT('Ctrl Pts',(-0.0266287903049468,-10.2963772509386,
10.4951080862604));
#11098=CARTESIAN_POINT('Ctrl Pts',(0.134388312888168,-10.2921837256933,
10.5253827273461));
#11099=CARTESIAN_POINT('Ctrl Pts',(0.430307821902681,-10.2767999672427,
10.6482195366313));
#11100=CARTESIAN_POINT('Ctrl Pts',(0.565223994153682,-10.2657970316571,
10.7407719255541));
#11101=CARTESIAN_POINT('Ctrl Pts',(0.778165371132575,-10.244422653795,10.9541478187001));
#11102=CARTESIAN_POINT('Ctrl Pts',(0.870426468860694,-10.232651025804,11.0892496287149));
#11103=CARTESIAN_POINT('Ctrl Pts',(0.992645040923687,-10.2141906775384,
11.3853937554379));
#11104=CARTESIAN_POINT('Ctrl Pts',(1.02259305653596,-10.2076973349447,11.5464521222423));
#11105=CARTESIAN_POINT('Ctrl Pts',(1.02228504001405,-10.2050778850534,11.6975542403122));
#11106=CARTESIAN_POINT('Ctrl Pts',(1.02197825097388,-10.2024688739752,11.8480541988248));
#11107=CARTESIAN_POINT('Ctrl Pts',(0.991604208232437,-10.2033604971208,
12.0085177147771));
#11108=CARTESIAN_POINT('Ctrl Pts',(0.868865917705535,-10.2115028582253,
12.3035493595844));
#11109=CARTESIAN_POINT('Ctrl Pts',(0.776506878336926,-10.2185593746734,
12.4381249833728));
#11110=CARTESIAN_POINT('Ctrl Pts',(0.563625112196363,-10.2324873030817,
12.6506454931746));
#11111=CARTESIAN_POINT('Ctrl Pts',(0.428839955813454,-10.2402603738984,
12.742790826072));
#11112=CARTESIAN_POINT('Ctrl Pts',(0.133477999031791,-10.2513527873625,
12.8650249475386));
#11113=CARTESIAN_POINT('Ctrl Pts',(-0.0271081339747381,-10.2544850951109,
12.8951080862604));
#11114=CARTESIAN_POINT('Ctrl Pts',(-0.177712466787678,-10.2544850951109,
12.8951080862604));
#11115=CARTESIAN_POINT('Origin',(-0.177712466787677,14.4000024114284,11.6951080862604));
#11116=CARTESIAN_POINT('',(-0.177712466787399,10.2963820737958,10.4951080862576));
#11117=CARTESIAN_POINT('',(-0.177712466787677,10.2544899179677,12.8951080862604));
#11118=CARTESIAN_POINT('Ctrl Pts',(-0.177712466787677,10.2963820737954,
10.4951080862604));
#11119=CARTESIAN_POINT('Ctrl Pts',(-0.328796143270408,10.2963820737954,
10.4951080862604));
#11120=CARTESIAN_POINT('Ctrl Pts',(-0.489813246463523,10.2921885485501,
10.5253827273461));
#11121=CARTESIAN_POINT('Ctrl Pts',(-0.785732755478036,10.2768047900996,
10.6482195366313));
#11122=CARTESIAN_POINT('Ctrl Pts',(-0.920648927729037,10.2658018545139,
10.7407719255541));
#11123=CARTESIAN_POINT('Ctrl Pts',(-1.13359030470793,10.2444274766519,10.9541478187001));
#11124=CARTESIAN_POINT('Ctrl Pts',(-1.22585140243605,10.2326558486608,11.0892496287149));
#11125=CARTESIAN_POINT('Ctrl Pts',(-1.34806997449904,10.2141955003952,11.3853937554379));
#11126=CARTESIAN_POINT('Ctrl Pts',(-1.37801799011132,10.2077021578015,11.5464521222423));
#11127=CARTESIAN_POINT('Ctrl Pts',(-1.37740318454924,10.202473696832,11.8480541988248));
#11128=CARTESIAN_POINT('Ctrl Pts',(-1.34702914180779,10.2033653199776,12.0085177147771));
#11129=CARTESIAN_POINT('Ctrl Pts',(-1.22429085128089,10.2115076810821,12.3035493595844));
#11130=CARTESIAN_POINT('Ctrl Pts',(-1.13193181191228,10.2185641975303,12.4381249833728));
#11131=CARTESIAN_POINT('Ctrl Pts',(-0.919050045771718,10.2324921259385,
12.6506454931746));
#11132=CARTESIAN_POINT('Ctrl Pts',(-0.78426488938881,10.2402651967552,12.742790826072));
#11133=CARTESIAN_POINT('Ctrl Pts',(-0.488902932607147,10.2513576102193,
12.8650249475386));
#11134=CARTESIAN_POINT('Ctrl Pts',(-0.328316799600617,10.2544899179677,
12.8951080862604));
#11135=CARTESIAN_POINT('Ctrl Pts',(-0.177712466787677,10.2544899179677,
12.8951080862604));
#11136=CARTESIAN_POINT('',(-0.177712466787678,6.00000241142841,12.8951080862604));
#11137=CARTESIAN_POINT('',(-0.177712466787678,14.4000024114284,12.8951080862604));
#11138=CARTESIAN_POINT('Origin',(-0.177712466787677,6.00000241142841,11.6951080862604));
#11139=CARTESIAN_POINT('Ctrl Pts',(-0.177712466787677,10.2544899179677,
12.8951080862604));
#11140=CARTESIAN_POINT('Ctrl Pts',(-0.0271081339747375,10.2544899179677,
12.8951080862604));
#11141=CARTESIAN_POINT('Ctrl Pts',(0.133477999031794,10.2513576102193,12.8650249475386));
#11142=CARTESIAN_POINT('Ctrl Pts',(0.428839955813457,10.2402651967552,12.742790826072));
#11143=CARTESIAN_POINT('Ctrl Pts',(0.563625112196364,10.2324921259385,12.6506454931746));
#11144=CARTESIAN_POINT('Ctrl Pts',(0.776506878336926,10.2185641975303,12.4381249833728));
#11145=CARTESIAN_POINT('Ctrl Pts',(0.868865917705535,10.2115076810821,12.3035493595844));
#11146=CARTESIAN_POINT('Ctrl Pts',(0.991604208232437,10.2033653199776,12.0085177147771));
#11147=CARTESIAN_POINT('Ctrl Pts',(1.02197825097388,10.202473696832,11.8480541988248));
#11148=CARTESIAN_POINT('Ctrl Pts',(1.02228504001405,10.2050827079102,11.6975542403122));
#11149=CARTESIAN_POINT('Ctrl Pts',(1.02259305653596,10.2077021578015,11.5464521222423));
#11150=CARTESIAN_POINT('Ctrl Pts',(0.992645040923687,10.2141955003952,11.3853937554379));
#11151=CARTESIAN_POINT('Ctrl Pts',(0.870426468860694,10.2326558486608,11.0892496287149));
#11152=CARTESIAN_POINT('Ctrl Pts',(0.778165371132575,10.2444274766519,10.9541478187001));
#11153=CARTESIAN_POINT('Ctrl Pts',(0.565223994153682,10.2658018545139,10.7407719255541));
#11154=CARTESIAN_POINT('Ctrl Pts',(0.43030782190268,10.2768047900996,10.6482195366313));
#11155=CARTESIAN_POINT('Ctrl Pts',(0.134388312888167,10.2921885485501,10.5253827273461));
#11156=CARTESIAN_POINT('Ctrl Pts',(-0.0266287903049473,10.2963820737954,
10.4951080862604));
#11157=CARTESIAN_POINT('Ctrl Pts',(-0.177712466787678,10.2963820737954,
10.4951080862604));
#11158=CARTESIAN_POINT('Origin',(-0.177712466787677,2.4114284077716E-6,
4.5587029190994));
#11159=CARTESIAN_POINT('',(8.03340298017176,-5.9999975885716,17.7536548280821));
#11160=CARTESIAN_POINT('',(8.03340298017176,6.00000241142841,17.7536548280823));
#11161=CARTESIAN_POINT('Origin',(-0.177712466787677,2.41142840473211E-6,
17.7536548280821));
#11162=CARTESIAN_POINT('',(8.07877050835459,6.00000241142841,15.6530982149009));
#11163=CARTESIAN_POINT('Ctrl Pts',(8.07877050835459,6.00000241142841,15.6530982149009));
#11164=CARTESIAN_POINT('Ctrl Pts',(8.06366240243391,6.00000241142841,16.3532840635641));
#11165=CARTESIAN_POINT('Ctrl Pts',(8.04853997260142,6.00000241142841,17.0534696033076));
#11166=CARTESIAN_POINT('Ctrl Pts',(8.03340298017176,6.00000241142841,17.7536548280823));
#11167=CARTESIAN_POINT('',(6.42417721261747,7.81192895720387,14.4149297172206));
#11168=CARTESIAN_POINT('Ctrl Pts',(6.42417721261747,7.81192895720387,14.4149297172206));
#11169=CARTESIAN_POINT('Ctrl Pts',(6.61539136987313,7.64482915707008,14.6557669349746));
#11170=CARTESIAN_POINT('Ctrl Pts',(6.84457822090961,7.43072762012922,14.8799697306037));
#11171=CARTESIAN_POINT('Ctrl Pts',(7.27350466710297,6.99326166671321,15.2278608961883));
#11172=CARTESIAN_POINT('Ctrl Pts',(7.52472544806286,6.71464397987196,15.3881604696605));
#11173=CARTESIAN_POINT('Ctrl Pts',(7.87311364932487,6.27809195147036,15.5649909889583));
#11174=CARTESIAN_POINT('Ctrl Pts',(7.97807672550604,6.13977704927159,15.6122830391166));
#11175=CARTESIAN_POINT('Ctrl Pts',(8.07877050835459,6.0000024114284,15.6530982149009));
#11176=CARTESIAN_POINT('',(4.37105054513769,9.20455838802752,12.1676472976633));
#11177=CARTESIAN_POINT('Ctrl Pts',(6.42417721261747,7.81192895720387,14.4149297172206));
#11178=CARTESIAN_POINT('Ctrl Pts',(5.80201464762526,8.35562949566307,13.6313062486766));
#11179=CARTESIAN_POINT('Ctrl Pts',(5.1062543034617,8.82759075958201,12.8682159131197));
#11180=CARTESIAN_POINT('Ctrl Pts',(4.37105054513769,9.20455838802752,12.1676472976633));
#11181=CARTESIAN_POINT('',(3.31160798786662,9.67660434821715,11.0613919569551));
#11182=CARTESIAN_POINT('Ctrl Pts',(3.31160798786662,9.67660434821715,11.0613919569551));
#11183=CARTESIAN_POINT('Ctrl Pts',(3.38725054660564,9.64772154529681,11.1479758305217));
#11184=CARTESIAN_POINT('Ctrl Pts',(3.46338662895692,9.61766757102202,11.2333252889551));
#11185=CARTESIAN_POINT('Ctrl Pts',(3.80017953593501,9.48013167695816,11.6032638240621));
#11186=CARTESIAN_POINT('Ctrl Pts',(4.08032391034575,9.35362526751858,11.8906166735587));
#11187=CARTESIAN_POINT('Ctrl Pts',(4.37105054513769,9.20455838802752,12.1676472976633));
#11188=CARTESIAN_POINT('',(-2.13351287620983,10.1557585661665,7.86054193760863));
#11189=CARTESIAN_POINT('Ctrl Pts',(3.31160798786662,9.67660434821715,11.0613919569551));
#11190=CARTESIAN_POINT('Ctrl Pts',(3.30666333464517,9.67849237853878,11.0557320845698));
#11191=CARTESIAN_POINT('Ctrl Pts',(3.3017142876189,9.68037750652116,11.0500800606398));
#11192=CARTESIAN_POINT('Ctrl Pts',(2.92188570807458,9.82470497845806,10.617283747585));
#11193=CARTESIAN_POINT('Ctrl Pts',(2.47116292610906,9.96831796451907,10.1818454164884));
#11194=CARTESIAN_POINT('Ctrl Pts',(1.4848560953238,10.1931375646734,9.40301401138184));
#11195=CARTESIAN_POINT('Ctrl Pts',(0.94889137476814,10.2728830446272,9.05968197552145));
#11196=CARTESIAN_POINT('Ctrl Pts',(-0.343612808630755,10.3610965901736,
8.38073343101154));
#11197=CARTESIAN_POINT('Ctrl Pts',(-1.23584670217506,10.3252285394421,8.051982603611));
#11198=CARTESIAN_POINT('Ctrl Pts',(-2.13351287620984,10.1557585661665,7.86054193760862));
#11199=CARTESIAN_POINT('',(-9.95140751249447,3.53610017282902,4.91934709248468));
#11200=CARTESIAN_POINT('Ctrl Pts',(-9.95140751249447,3.53610017282902,4.91934709248468));
#11201=CARTESIAN_POINT('Ctrl Pts',(-9.89707498092324,3.68471646024097,4.94970641657277));
#11202=CARTESIAN_POINT('Ctrl Pts',(-9.83935880934888,3.8319721919242,4.98171908114857));
#11203=CARTESIAN_POINT('Ctrl Pts',(-9.24965882931434,5.24053783544831,5.30577915095143));
#11204=CARTESIAN_POINT('Ctrl Pts',(-8.46376367800013,6.37827852692683,5.71189719320963));
#11205=CARTESIAN_POINT('Ctrl Pts',(-6.65732758822298,8.19454584161434,6.50688309595488));
#11206=CARTESIAN_POINT('Ctrl Pts',(-5.49960232856536,8.99469099268257,6.9534533168386));
#11207=CARTESIAN_POINT('Ctrl Pts',(-3.54725844985039,9.81102690694312,7.52942979311924));
#11208=CARTESIAN_POINT('Ctrl Pts',(-2.84446760524541,10.0215377584598,7.70892026491894));
#11209=CARTESIAN_POINT('Ctrl Pts',(-2.13351287620983,10.1557585661665,7.86054193760862));
#11210=CARTESIAN_POINT('',(-9.86226050887947,3.53610097918737,9.71934528208445));
#11211=CARTESIAN_POINT('Ctrl Pts',(-9.95140898508777,3.53610097918737,4.91934626964542));
#11212=CARTESIAN_POINT('Ctrl Pts',(-9.93632582125981,3.53610097918737,5.73181939317775));
#11213=CARTESIAN_POINT('Ctrl Pts',(-9.92124034862481,3.53610097918737,6.54429346176475));
#11214=CARTESIAN_POINT('Ctrl Pts',(-9.90615078043081,3.53610097918737,7.35676745427743));
#11215=CARTESIAN_POINT('Ctrl Pts',(-9.89152455533496,3.53610097918737,8.14429346868886));
#11216=CARTESIAN_POINT('Ctrl Pts',(-9.87689448233653,3.53610097918737,8.93181941162615));
#11217=CARTESIAN_POINT('Ctrl Pts',(-9.86226050887948,3.53610097918737,9.71934528208445));
#11218=CARTESIAN_POINT('',(-10.4876331192705,2.4114284090342E-6,9.71934528208445));
#11219=CARTESIAN_POINT('Origin',(-0.177712466787677,2.4114284077716E-6,
9.71934528208445));
#11220=CARTESIAN_POINT('',(-10.1203897656684,2.41142840880554E-6,30.7587029190994));
#11221=CARTESIAN_POINT('',(-10.5777124667877,2.41142840904524E-6,4.5587029190994));
#11222=CARTESIAN_POINT('',(9.76497550923372,2.41142840604871E-6,30.7580912261184));
#11223=CARTESIAN_POINT('Ctrl Pts',(-10.1203897656684,2.41142840862185E-6,
30.7587029190994));
#11224=CARTESIAN_POINT('Ctrl Pts',(-10.1203897656684,1.27089668043473,30.7587029190994));
#11225=CARTESIAN_POINT('Ctrl Pts',(-9.86008094032418,2.6077169391002,30.9068158434723));
#11226=CARTESIAN_POINT('Ctrl Pts',(-8.83558352698103,5.04135256634328,31.4099925598972));
#11227=CARTESIAN_POINT('Ctrl Pts',(-8.07213111882965,6.14055961719644,31.7549337629918));
#11228=CARTESIAN_POINT('Ctrl Pts',(-6.32709993360833,7.87313335557606,32.3805754170083));
#11229=CARTESIAN_POINT('Ctrl Pts',(-5.22311287806905,8.62972184841935,32.7057628801753));
#11230=CARTESIAN_POINT('Ctrl Pts',(-2.78235121183544,9.64293330397286,33.1623258591164));
#11231=CARTESIAN_POINT('Ctrl Pts',(-1.44421313614939,9.89851844327917,33.2887002128102));
#11232=CARTESIAN_POINT('Ctrl Pts',(1.08880241943988,9.8985196265464,33.2886324234761));
#11233=CARTESIAN_POINT('Ctrl Pts',(2.4269477644944,9.64293055183899,33.1621838232405));
#11234=CARTESIAN_POINT('Ctrl Pts',(4.86771468168172,8.62971246476211,32.7054793231542));
#11235=CARTESIAN_POINT('Ctrl Pts',(5.97170006728986,7.87312153584118,32.3802243211076));
#11236=CARTESIAN_POINT('Ctrl Pts',(7.71672174055816,6.14055081828832,31.7544717166664));
#11237=CARTESIAN_POINT('Ctrl Pts',(8.48016993081502,5.04134981420114,31.409478412752));
#11238=CARTESIAN_POINT('Ctrl Pts',(9.50466493926388,2.60772113563203,30.9062263543421));
#11239=CARTESIAN_POINT('Ctrl Pts',(9.76497550923372,1.27090121854302,30.7580912261184));
#11240=CARTESIAN_POINT('Ctrl Pts',(9.76497550923372,2.41142840889941E-6,
30.7580912261184));
#11241=CARTESIAN_POINT('Ctrl Pts',(9.76497550923372,2.41142840751163E-6,
30.7580912261184));
#11242=CARTESIAN_POINT('Ctrl Pts',(9.76497550923372,-1.2708963956862,30.7580912261184));
#11243=CARTESIAN_POINT('Ctrl Pts',(9.50466493926388,-2.60771631277522,30.9062263543421));
#11244=CARTESIAN_POINT('Ctrl Pts',(8.48016993081501,-5.04134499134433,31.409478412752));
#11245=CARTESIAN_POINT('Ctrl Pts',(7.71672174055816,-6.14054599543151,31.7544717166664));
#11246=CARTESIAN_POINT('Ctrl Pts',(5.97170006728986,-7.87311671298437,32.3802243211076));
#11247=CARTESIAN_POINT('Ctrl Pts',(4.86771468168172,-8.62970764190529,32.7054793231542));
#11248=CARTESIAN_POINT('Ctrl Pts',(2.4269477644944,-9.64292572898218,33.1621838232405));
#11249=CARTESIAN_POINT('Ctrl Pts',(1.08880241943988,-9.89851480368958,33.2886324234761));
#11250=CARTESIAN_POINT('Ctrl Pts',(-1.44421313614939,-9.89851362042235,
33.2887002128102));
#11251=CARTESIAN_POINT('Ctrl Pts',(-2.78235121183544,-9.64292848111604,
33.1623258591164));
#11252=CARTESIAN_POINT('Ctrl Pts',(-5.22311287806905,-8.62971702556254,
32.7057628801753));
#11253=CARTESIAN_POINT('Ctrl Pts',(-6.32709993360833,-7.87312853271924,
32.3805754170083));
#11254=CARTESIAN_POINT('Ctrl Pts',(-8.07213111882965,-6.14055479433963,
31.7549337629918));
#11255=CARTESIAN_POINT('Ctrl Pts',(-8.83558352698103,-5.04134774348647,
31.4099925598972));
#11256=CARTESIAN_POINT('Ctrl Pts',(-9.86008094032418,-2.60771211624338,
30.9068158434723));
#11257=CARTESIAN_POINT('Ctrl Pts',(-10.1203897656684,-1.27089185757792,
30.7587029190994));
#11258=CARTESIAN_POINT('Ctrl Pts',(-10.1203897656684,2.41142840695652E-6,
30.7587029190994));
#11259=CARTESIAN_POINT('',(-9.86226050887947,-3.53609615633055,9.71934528208445));
#11260=CARTESIAN_POINT('Origin',(-0.177712466787677,2.4114284077716E-6,
9.71934528208445));
#11261=CARTESIAN_POINT('',(-9.95140789577959,-3.53609567260447,4.91934619906695));
#11262=CARTESIAN_POINT('Ctrl Pts',(-9.86226050887948,-3.53609615633055,
9.71934528208445));
#11263=CARTESIAN_POINT('Ctrl Pts',(-9.87689448233653,-3.53609615633055,
8.93181941162615));
#11264=CARTESIAN_POINT('Ctrl Pts',(-9.89152455533695,-3.53609615633055,
8.14429346867934));
#11265=CARTESIAN_POINT('Ctrl Pts',(-9.90615078043284,-3.53609615633055,
7.35676745426777));
#11266=CARTESIAN_POINT('Ctrl Pts',(-9.92124034862687,-3.53609615633055,
6.54429346175493));
#11267=CARTESIAN_POINT('Ctrl Pts',(-9.93632582125982,-3.53609615633055,
5.73181939317775));
#11268=CARTESIAN_POINT('Ctrl Pts',(-9.95140898508777,-3.53609615633055,
4.91934626964541));
#11269=CARTESIAN_POINT('',(-2.13351287620984,-10.1557537433096,7.86054193760862));
#11270=CARTESIAN_POINT('Ctrl Pts',(-2.13351287620984,-10.1557537433096,
7.86054193760862));
#11271=CARTESIAN_POINT('Ctrl Pts',(-2.84446760524542,-10.021532935603,7.70892026491893));
#11272=CARTESIAN_POINT('Ctrl Pts',(-3.54725844985039,-9.8110220840863,7.52942979311924));
#11273=CARTESIAN_POINT('Ctrl Pts',(-5.49960232856536,-8.99468616982575,
6.9534533168386));
#11274=CARTESIAN_POINT('Ctrl Pts',(-6.65732758822298,-8.19454101875751,
6.50688309595488));
#11275=CARTESIAN_POINT('Ctrl Pts',(-8.46376367800012,-6.37827370407001,
5.71189719320963));
#11276=CARTESIAN_POINT('Ctrl Pts',(-9.24965882931434,-5.2405330125915,5.30577915095143));
#11277=CARTESIAN_POINT('Ctrl Pts',(-9.83935880934888,-3.83196736906738,
4.98171908114857));
#11278=CARTESIAN_POINT('Ctrl Pts',(-9.89707498092324,-3.68471163738415,
4.94970641657277));
#11279=CARTESIAN_POINT('Ctrl Pts',(-9.95140751249447,-3.5360953499722,4.91934709248468));
#11280=CARTESIAN_POINT('',(3.31160798786661,-9.67659952536034,11.0613919569551));
#11281=CARTESIAN_POINT('Ctrl Pts',(-2.13351287620984,-10.1557537433096,
7.86054193760862));
#11282=CARTESIAN_POINT('Ctrl Pts',(-1.23584670217506,-10.3252237165853,
8.051982603611));
#11283=CARTESIAN_POINT('Ctrl Pts',(-0.343612808630755,-10.3610917673168,
8.38073343101154));
#11284=CARTESIAN_POINT('Ctrl Pts',(0.948891374768143,-10.2728782217704,
9.05968197552145));
#11285=CARTESIAN_POINT('Ctrl Pts',(1.48485609532381,-10.1931327418166,9.40301401138184));
#11286=CARTESIAN_POINT('Ctrl Pts',(2.47116292610906,-9.96831314166225,10.1818454164884));
#11287=CARTESIAN_POINT('Ctrl Pts',(2.92188570807458,-9.82470015560125,10.617283747585));
#11288=CARTESIAN_POINT('Ctrl Pts',(3.3017142876189,-9.68037268366434,11.0500800606398));
#11289=CARTESIAN_POINT('Ctrl Pts',(3.30666333464517,-9.67848755568196,11.0557320845698));
#11290=CARTESIAN_POINT('Ctrl Pts',(3.31160798786662,-9.67659952536034,11.0613919569551));
#11291=CARTESIAN_POINT('',(4.37105054513769,-9.2045535651707,12.1676472976633));
#11292=CARTESIAN_POINT('Ctrl Pts',(4.37105054513769,-9.2045535651707,12.1676472976633));
#11293=CARTESIAN_POINT('Ctrl Pts',(4.08032391034576,-9.35362044466177,11.8906166735587));
#11294=CARTESIAN_POINT('Ctrl Pts',(3.80017953593501,-9.48012685410135,11.6032638240621));
#11295=CARTESIAN_POINT('Ctrl Pts',(3.46338662895692,-9.6176627481652,11.2333252889551));
#11296=CARTESIAN_POINT('Ctrl Pts',(3.38725054660564,-9.64771672243999,11.1479758305217));
#11297=CARTESIAN_POINT('Ctrl Pts',(3.31160798786662,-9.67659952536034,11.0613919569551));
#11298=CARTESIAN_POINT('',(6.42417721261744,-7.81192413434708,14.4149297172206));
#11299=CARTESIAN_POINT('Ctrl Pts',(4.37105054513769,-9.2045535651707,12.1676472976633));
#11300=CARTESIAN_POINT('Ctrl Pts',(5.10619880095024,-8.82761439502656,12.8681630253085));
#11301=CARTESIAN_POINT('Ctrl Pts',(5.80196171161444,-8.3556709329627,13.6312395749441));
#11302=CARTESIAN_POINT('Ctrl Pts',(6.42417721261744,-7.81192413434708,14.4149297172206));
#11303=CARTESIAN_POINT('',(8.07877050835458,-5.9999975885716,15.6530982149009));
#11304=CARTESIAN_POINT('Ctrl Pts',(8.07877050835458,-5.9999975885716,15.6530982149009));
#11305=CARTESIAN_POINT('Ctrl Pts',(7.97807672550604,-6.13977222641478,15.6122830391166));
#11306=CARTESIAN_POINT('Ctrl Pts',(7.87311364932487,-6.27808712861355,15.5649909889583));
#11307=CARTESIAN_POINT('Ctrl Pts',(7.52472544806286,-6.71463915701515,15.3881604696605));
#11308=CARTESIAN_POINT('Ctrl Pts',(7.27350466710297,-6.9932568438564,15.2278608961883));
#11309=CARTESIAN_POINT('Ctrl Pts',(6.8445782209096,-7.43072279727242,14.8799697306037));
#11310=CARTESIAN_POINT('Ctrl Pts',(6.6153913698731,-7.64482433421329,14.6557669349745));
#11311=CARTESIAN_POINT('Ctrl Pts',(6.42417721261744,-7.81192413434708,14.4149297172206));
#11312=CARTESIAN_POINT('Ctrl Pts',(8.03340298017176,-5.9999975885716,17.7536548280821));
#11313=CARTESIAN_POINT('Ctrl Pts',(8.04853997260142,-5.9999975885716,17.0534696033075));
#11314=CARTESIAN_POINT('Ctrl Pts',(8.0636624024339,-5.9999975885716,16.353284063564));
#11315=CARTESIAN_POINT('Ctrl Pts',(8.07877050835458,-5.9999975885716,15.6530982149009));
#11316=CARTESIAN_POINT('Origin',(15.9282673556341,20.,0.0390576814896602));
#11317=CARTESIAN_POINT('',(4.37105054513769,6.00000241142841,12.1676472976633));
#11318=CARTESIAN_POINT('',(4.37105054513769,20.,12.1676472976633));
#11319=CARTESIAN_POINT('',(3.31160798786661,6.00000241142841,11.0613919569551));
#11320=CARTESIAN_POINT('Origin',(15.9282673556341,6.00000241142841,0.0390576814896602));
#11321=CARTESIAN_POINT('',(3.31160798786661,20.,11.0613919569551));
#11322=CARTESIAN_POINT('Origin',(15.9282673556341,20.,0.0390576814896602));
#11323=CARTESIAN_POINT('',(4.37105054513769,-5.99999758857159,12.1676472976633));
#11324=CARTESIAN_POINT('',(3.31160798786661,-5.99999758857159,11.0613919569551));
#11325=CARTESIAN_POINT('Origin',(15.9282673556341,-5.99999758857159,0.0390576814896602));
#11326=CARTESIAN_POINT('',(4.37105054513769,20.,12.1676472976633));
#11327=CARTESIAN_POINT('',(3.31160798786661,20.,11.0613919569551));
#11328=CARTESIAN_POINT('Origin',(-0.177712466787677,2.41142840473615E-6,
17.7187500152076));
#11329=CARTESIAN_POINT('',(5.36743577950585,6.00000241142841,15.7187500152076));
#11330=CARTESIAN_POINT('',(5.36743577950585,-5.9999975885716,15.7187500152076));
#11331=CARTESIAN_POINT('Origin',(-0.177712466787677,2.41142840496745E-6,
15.7187500152076));
#11332=CARTESIAN_POINT('Ctrl Pts',(8.03340298017176,6.00000241142841,17.7536548280823));
#11333=CARTESIAN_POINT('Ctrl Pts',(8.0336564955911,6.00000241142841,17.7419280764372));
#11334=CARTESIAN_POINT('Ctrl Pts',(8.03378024422029,6.00000241142841,17.7302885973412));
#11335=CARTESIAN_POINT('Ctrl Pts',(8.03378024422029,6.00000241142841,17.7187500152076));
#11336=CARTESIAN_POINT('Ctrl Pts',(8.03378024422029,6.00000241142841,17.4922929238556));
#11337=CARTESIAN_POINT('Ctrl Pts',(7.97327314315844,6.00000241142841,17.2273662487111));
#11338=CARTESIAN_POINT('Ctrl Pts',(7.77162808002468,6.00000241142841,16.7923068382797));
#11339=CARTESIAN_POINT('Ctrl Pts',(7.58483347292422,6.00000241142841,16.552880331799));
#11340=CARTESIAN_POINT('Ctrl Pts',(7.16867991474912,6.00000241142841,16.187909747159));
#11341=CARTESIAN_POINT('Ctrl Pts',(6.85309265217151,6.00000241142841,16.0135423105674));
#11342=CARTESIAN_POINT('Ctrl Pts',(6.20801832838943,6.00000241142841,15.7841079557633));
#11343=CARTESIAN_POINT('Ctrl Pts',(5.75163519004221,6.00000241142841,15.7187500152076));
#11344=CARTESIAN_POINT('Ctrl Pts',(5.36743577950585,6.00000241142841,15.7187500152076));
#11345=CARTESIAN_POINT('Ctrl Pts',(5.36743577950585,-5.9999975885716,15.7187500152076));
#11346=CARTESIAN_POINT('Ctrl Pts',(5.72647842293398,-5.9999975885716,15.7187500152076));
#11347=CARTESIAN_POINT('Ctrl Pts',(6.15352297661853,-5.9999975885716,15.7758961583859));
#11348=CARTESIAN_POINT('Ctrl Pts',(6.76579277314527,-5.9999975885716,15.9756283261255));
#11349=CARTESIAN_POINT('Ctrl Pts',(7.07130289664905,-5.9999975885716,16.1292918308475));
#11350=CARTESIAN_POINT('Ctrl Pts',(7.51408278212533,-5.9999975885716,16.4745709963669));
#11351=CARTESIAN_POINT('Ctrl Pts',(7.73059566582944,-5.9999975885716,16.7260080521206));
#11352=CARTESIAN_POINT('Ctrl Pts',(7.96379246621659,-5.9999975885716,17.1910498696455));
#11353=CARTESIAN_POINT('Ctrl Pts',(8.03378024422029,-5.9999975885716,17.4750238564616));
#11354=CARTESIAN_POINT('Ctrl Pts',(8.03378024422029,-5.9999975885716,17.7187500152076));
#11355=CARTESIAN_POINT('Ctrl Pts',(8.03378024422029,-5.9999975885716,17.7302885973412));
#11356=CARTESIAN_POINT('Ctrl Pts',(8.03365649559111,-5.9999975885716,17.741928076437));
#11357=CARTESIAN_POINT('Ctrl Pts',(8.03340298017176,-5.9999975885716,17.7536548280821));
#11358=CARTESIAN_POINT('',(8.34339394095876,2.41142818149586E-6,15.7498126454214));
#11359=CARTESIAN_POINT('Ctrl Pts',(8.70260319627842,2.41142840359115E-6,
15.8491426817344));
#11360=CARTESIAN_POINT('Ctrl Pts',(8.70260319627842,0.1457045944121,15.8491426817344));
#11361=CARTESIAN_POINT('Ctrl Pts',(8.69364580031477,0.296936499486973,15.8471441058903));
#11362=CARTESIAN_POINT('Ctrl Pts',(8.65874844698062,0.550908277238344,15.8389323814439));
#11363=CARTESIAN_POINT('Ctrl Pts',(8.63853053418753,0.646402965673418,15.8340793094607));
#11364=CARTESIAN_POINT('Ctrl Pts',(8.60408557717993,0.759711181045861,15.8254316219397));
#11365=CARTESIAN_POINT('Ctrl Pts',(8.5850108075902,0.815595445147395,15.8206049324342));
#11366=CARTESIAN_POINT('Ctrl Pts',(8.55163815579824,0.871468558310266,15.8117236803648));
#11367=CARTESIAN_POINT('Ctrl Pts',(8.54152593085035,0.885874415477635,15.8090050962758));
#11368=CARTESIAN_POINT('Ctrl Pts',(8.52435773636745,0.901956274035506,15.8042960825429));
#11369=CARTESIAN_POINT('Ctrl Pts',(8.51797517577937,0.906754467657781,15.8025322161507));
#11370=CARTESIAN_POINT('Ctrl Pts',(8.50624686619019,0.912133938580912,15.7992540736978));
#11371=CARTESIAN_POINT('Ctrl Pts',(8.50122322934824,0.91355243852032,15.7978404300894));
#11372=CARTESIAN_POINT('Ctrl Pts',(8.49091881899635,0.91416086088759,15.7949175385542));
#11373=CARTESIAN_POINT('Ctrl Pts',(8.48596709871937,0.913383948477207,15.7935022066964));
#11374=CARTESIAN_POINT('Ctrl Pts',(8.474893845048,0.909319390924804,15.7903156787572));
#11375=CARTESIAN_POINT('Ctrl Pts',(8.46924834293951,0.905476072857559,15.7886748573832));
#11376=CARTESIAN_POINT('Ctrl Pts',(8.45591203444658,0.893350354530391,15.7847743670347));
#11377=CARTESIAN_POINT('Ctrl Pts',(8.44886017802113,0.883355752885808,15.7826834861937));
#11378=CARTESIAN_POINT('Ctrl Pts',(8.42921811137653,0.849625584159388,15.7768229351228));
#11379=CARTESIAN_POINT('Ctrl Pts',(8.41857418536194,0.818832096261853,15.77357085887));
#11380=CARTESIAN_POINT('Ctrl Pts',(8.38963278923615,0.718049400748019,15.7646736905908));
#11381=CARTESIAN_POINT('Ctrl Pts',(8.37640202783079,0.623503318149914,15.7604475541772));
#11382=CARTESIAN_POINT('Ctrl Pts',(8.35677624531277,0.44067682070463,15.7541764262857));
#11383=CARTESIAN_POINT('Ctrl Pts',(8.35027668860286,0.325088164238925,15.7520555912301));
#11384=CARTESIAN_POINT('Ctrl Pts',(8.34306653761666,0.101377390155308,15.7497077216999));
#11385=CARTESIAN_POINT('Ctrl Pts',(8.34243149243459,-0.0207353219056583,
15.7494989245869));
#11386=CARTESIAN_POINT('Ctrl Pts',(8.34693351311756,-0.248426106820748,
15.7509676266811));
#11387=CARTESIAN_POINT('Ctrl Pts',(8.35201202114988,-0.366559655312288,
15.7526295432987));
#11388=CARTESIAN_POINT('Ctrl Pts',(8.3687589044063,-0.562240685563907,15.7580128828001));
#11389=CARTESIAN_POINT('Ctrl Pts',(8.38041238916994,-0.663093948738599,
15.7617584461812));
#11390=CARTESIAN_POINT('Ctrl Pts',(8.40759738858707,-0.783137084891655,
15.7702044457537));
#11391=CARTESIAN_POINT('Ctrl Pts',(8.41958541271743,-0.826709692526858,
15.7739090533259));
#11392=CARTESIAN_POINT('Ctrl Pts',(8.44203546065897,-0.87243390895032,15.7806521090902));
#11393=CARTESIAN_POINT('Ctrl Pts',(8.44958624407923,-0.885261390162398,
15.782905772264));
#11394=CARTESIAN_POINT('Ctrl Pts',(8.46336792824719,-0.900507134123406,
15.7869579908969));
#11395=CARTESIAN_POINT('Ctrl Pts',(8.46876320763649,-0.905270445033883,
15.788535226918));
#11396=CARTESIAN_POINT('Ctrl Pts',(8.47924099692529,-0.911158565852659,
15.7915688525739));
#11397=CARTESIAN_POINT('Ctrl Pts',(8.48394623004557,-0.912880662985735,
15.792923034465));
#11398=CARTESIAN_POINT('Ctrl Pts',(8.49406517207035,-0.914291240571678,
15.7958131414122));
#11399=CARTESIAN_POINT('Ctrl Pts',(8.49915094354501,-0.913869835331626,
15.7972547181197));
#11400=CARTESIAN_POINT('Ctrl Pts',(8.51110380005296,-0.91053442442188,15.800618271558));
#11401=CARTESIAN_POINT('Ctrl Pts',(8.51754939660892,-0.906818762271611,
15.8024119432661));
#11402=CARTESIAN_POINT('Ctrl Pts',(8.53354825296255,-0.894484934836979,
15.806829539192));
#11403=CARTESIAN_POINT('Ctrl Pts',(8.54261523602715,-0.883575448092069,
15.8092896800772));
#11404=CARTESIAN_POINT('Ctrl Pts',(8.57970306582927,-0.830473956918792,
15.8192582016274));
#11405=CARTESIAN_POINT('Ctrl Pts',(8.60192499259373,-0.766124180642222,
15.8248840078164));
#11406=CARTESIAN_POINT('Ctrl Pts',(8.63698938385199,-0.65269060197119,15.8337015828562));
#11407=CARTESIAN_POINT('Ctrl Pts',(8.65729303891214,-0.558598640774244,
15.8385845860059));
#11408=CARTESIAN_POINT('Ctrl Pts',(8.69327905844745,-0.303189203914345,
15.8470644051406));
#11409=CARTESIAN_POINT('Ctrl Pts',(8.70260319627842,-0.148645966954802,
15.8491426817344));
#11410=CARTESIAN_POINT('Ctrl Pts',(8.70260319627842,2.41142840350442E-6,
15.8491426817344));
#11411=CARTESIAN_POINT('Origin',(3.70657129686984,28.8000024114284,-19.5236399353513));
#11412=CARTESIAN_POINT('',(-6.57771246678768,-5.99999758857159,6.51927671137959));
#11413=CARTESIAN_POINT('',(-2.13351287620984,-5.9999975885716,7.86054193760862));
#11414=CARTESIAN_POINT('Origin',(3.70657129686984,-5.99999758857159,-19.5236399353513));
#11415=CARTESIAN_POINT('',(-2.13351287620984,28.8000024114284,7.86054193760862));
#11416=CARTESIAN_POINT('Ctrl Pts',(-9.95140751249447,-3.53609534997221,
4.91934709248468));
#11417=CARTESIAN_POINT('Ctrl Pts',(-10.368177467718,-2.39610055019092,4.68646903996433));
#11418=CARTESIAN_POINT('Ctrl Pts',(-10.5777124667877,-1.17144708556741,
4.5587029190994));
#11419=CARTESIAN_POINT('Ctrl Pts',(-10.5777124667877,1.17145190842423,4.5587029190994));
#11420=CARTESIAN_POINT('Ctrl Pts',(-10.368177467718,2.39610537304773,4.68646903996433));
#11421=CARTESIAN_POINT('Ctrl Pts',(-9.95140751249447,3.53610017282902,4.91934709248468));
#11422=CARTESIAN_POINT('',(-2.13351287620984,6.00000241142841,7.86054193760862));
#11423=CARTESIAN_POINT('',(-2.13351287620984,28.8000024114284,7.86054193760862));
#11424=CARTESIAN_POINT('',(-6.57771246678768,6.00000241142841,6.51927671137958));
#11425=CARTESIAN_POINT('Origin',(3.70657129686984,6.00000241142841,-19.5236399353513));
#11426=CARTESIAN_POINT('',(-6.57771246678768,28.8000024114284,6.51927671137959));
#11427=CARTESIAN_POINT('Origin',(-9.15718923943328,2.4114284077716E-6,-4.42077385354621));
#11428=CARTESIAN_POINT('',(-15.1031958253685,-3.53609615633055,1.52523273238902));
#11429=CARTESIAN_POINT('',(-16.37182497547,-3.53609615633055,2.79386188249054));
#11430=CARTESIAN_POINT('',(-14.5375104004193,-3.53609615633055,0.959547307439778));
#11431=CARTESIAN_POINT('',(-16.37182497547,-1.99999758857159,2.79386188249054));
#11432=CARTESIAN_POINT('',(-16.37182497547,-1.99999758857159,2.79386188249054));
#11433=CARTESIAN_POINT('',(-15.1031958253685,-1.99999758857159,1.52523273238902));
#11434=CARTESIAN_POINT('',(-9.15718923943328,-1.99999758857159,-4.42077385354621));
#11435=CARTESIAN_POINT('',(-15.1031958253685,-3.53609615633055,1.52523273238902));
#11436=CARTESIAN_POINT('Origin',(-0.177712466787677,2.4114284077716E-6,
4.5587029190994));
#11437=CARTESIAN_POINT('Origin',(-0.177712466787677,2.4114284077716E-6,
4.91934528208444));
#11438=CARTESIAN_POINT('Origin',(-0.17826912272476,28.8000024114284,12.4886663257821));
#11439=CARTESIAN_POINT('',(5.77713238753779,-3.53609615633055,32.417870847076));
#11440=CARTESIAN_POINT('',(5.77713238753779,3.53610097918737,32.417870847076));
#11441=CARTESIAN_POINT('',(5.77713238753779,28.8000024114284,32.417870847076));
#11442=CARTESIAN_POINT('',(-6.13255732111315,-3.53609615633055,32.4182035018063));
#11443=CARTESIAN_POINT('Origin',(-0.17826912272476,-3.53609615633055,12.4886663257821));
#11444=CARTESIAN_POINT('',(-6.13255732111315,3.53610097918737,32.4182035018063));
#11445=CARTESIAN_POINT('',(-6.13255732111315,28.8000024114284,32.4182035018063));
#11446=CARTESIAN_POINT('Origin',(-0.17826912272476,3.53610097918737,12.4886663257821));
#11447=CARTESIAN_POINT('Origin',(12.6222875332123,6.00000241142841,15.7187500152076));
#11448=CARTESIAN_POINT('',(-6.57771246678768,-5.9999975885716,15.7187500152076));
#11449=CARTESIAN_POINT('',(12.6222875332123,-5.9999975885716,15.7187500152076));
#11450=CARTESIAN_POINT('',(-6.57771246678768,6.00000241142841,15.7187500152076));
#11451=CARTESIAN_POINT('',(-6.57771246678768,6.00000241142841,15.7187500152076));
#11452=CARTESIAN_POINT('',(12.6222875332123,6.00000241142841,15.7187500152076));
#11453=CARTESIAN_POINT('Origin',(12.6222875332123,-5.99999758857159,-6.60134417700877));
#11454=CARTESIAN_POINT('',(6.42417721261744,-5.9999975885716,14.4149297172206));
#11455=CARTESIAN_POINT('Origin',(9.60397861284329,-5.9999975885716,11.8903072744979));
#11456=CARTESIAN_POINT('Origin',(-10.8056176096432,-5.9999975885716,28.0946289238114));
#11457=CARTESIAN_POINT('Origin',(-4.21925722373829,-5.9999975885716,17.6406068922372));
#11458=CARTESIAN_POINT('',(-6.57771246678768,-5.99999758857159,-6.60134417700877));
#11459=CARTESIAN_POINT('Origin',(12.6222875332123,6.00000241142841,-6.60134417700877));
#11460=CARTESIAN_POINT('',(6.42417721261744,6.00000241142841,14.4149297172206));
#11461=CARTESIAN_POINT('Origin',(-10.8056176096432,6.0000024114284,28.0946289238114));
#11462=CARTESIAN_POINT('Origin',(9.60397861284329,6.00000241142841,11.8903072744979));
#11463=CARTESIAN_POINT('',(-6.57771246678768,6.00000241142841,-6.60134417700877));
#11464=CARTESIAN_POINT('Origin',(-4.21925722373829,6.0000024114284,17.6406068922372));
#11465=CARTESIAN_POINT('Origin',(-6.57771246678768,2.4114284077716E-6,4.5587029190994));
#11466=CARTESIAN_POINT('Origin',(10.4270144578429,-3.53609615633055,4.91934528208444));
#11467=CARTESIAN_POINT('',(-10.5777124257746,-3.53609615633055,4.91934528208445));
#11468=CARTESIAN_POINT('',(10.4270144578429,-3.53609615633055,4.91934528208444));
#11469=CARTESIAN_POINT('',(-10.5777124257746,3.53610097918737,4.91934528208445));
#11470=CARTESIAN_POINT('',(-10.5777124257746,-3.53609615633055,4.91934528208444));
#11471=CARTESIAN_POINT('',(10.4270144578429,3.53610097918737,4.91934528208444));
#11472=CARTESIAN_POINT('Origin',(10.4270144578429,3.53610097918737,9.71934528208445));
#11473=CARTESIAN_POINT('',(-16.37182497547,3.53610097918737,2.79386188249054));
#11474=CARTESIAN_POINT('',(-15.1031958253685,3.53610097918737,1.52523273238902));
#11475=CARTESIAN_POINT('',(-16.9375104004193,3.53610097918737,3.35954730743978));
#11476=CARTESIAN_POINT('',(-16.37182497547,3.53610097918737,3.92523273238902));
#11477=CARTESIAN_POINT('Origin',(-15.8061395505208,3.53610097918737,3.35954730743978));
#11478=CARTESIAN_POINT('',(-10.5777124257746,3.53610097918737,9.71934528208445));
#11479=CARTESIAN_POINT('',(-16.9375104004193,3.53610097918737,3.35954730743978));
#11480=CARTESIAN_POINT('',(10.4270144578429,3.53610097918737,9.71934528208445));
#11481=CARTESIAN_POINT('',(-13.97182497547,3.53610097918737,1.52523273238902));
#11482=CARTESIAN_POINT('',(-14.5375104004193,3.53610097918737,0.959547307439778));
#11483=CARTESIAN_POINT('Origin',(-14.5375104004193,3.53610097918737,2.09091815733826));
#11484=CARTESIAN_POINT('Origin',(10.4270144578429,-3.53609615633055,9.71934528208445));
#11485=CARTESIAN_POINT('',(-10.5777124257746,-3.53609615633055,9.71934528208445));
#11486=CARTESIAN_POINT('',(-10.5777124257746,-3.53609615633055,9.71934528208445));
#11487=CARTESIAN_POINT('',(10.4270144578429,-3.53609615633055,9.71934528208445));
#11488=CARTESIAN_POINT('Origin',(10.4270144578429,-3.53609615633055,9.71934528208445));
#11489=CARTESIAN_POINT('',(-16.37182497547,-3.53609615633055,3.92523273238902));
#11490=CARTESIAN_POINT('',(-16.9375104004193,-3.53609615633055,3.35954730743978));
#11491=CARTESIAN_POINT('Origin',(-15.8061395505208,-3.53609615633055,3.35954730743978));
#11492=CARTESIAN_POINT('',(-13.97182497547,-3.53609615633055,1.52523273238902));
#11493=CARTESIAN_POINT('Origin',(-14.5375104004193,-3.53609615633055,2.09091815733826));
#11494=CARTESIAN_POINT('',(-14.5375104004193,-3.53609615633055,0.959547307439778));
#11495=CARTESIAN_POINT('Origin',(-14.5375104004193,3.53610097918737,0.959547307439778));
#11496=CARTESIAN_POINT('',(-13.97182497547,-1.99999758857159,1.52523273238902));
#11497=CARTESIAN_POINT('',(-13.97182497547,-1.99999758857159,1.52523273238902));
#11498=CARTESIAN_POINT('',(-11.1433978507238,-1.99999758857159,4.3536598571352));
#11499=CARTESIAN_POINT('',(-14.5375104004193,-1.99999758857159,0.959547307439778));
#11500=CARTESIAN_POINT('',(-11.1433978507238,2.00000241142841,4.35365985713521));
#11501=CARTESIAN_POINT('',(-11.1433978507238,3.53610097918737,4.3536598571352));
#11502=CARTESIAN_POINT('',(-13.97182497547,2.00000241142841,1.52523273238902));
#11503=CARTESIAN_POINT('',(-14.5375104004193,2.00000241142841,0.959547307439778));
#11504=CARTESIAN_POINT('',(-13.97182497547,3.53610097918737,1.52523273238902));
#11505=CARTESIAN_POINT('Origin',(-16.9375104004193,-3.53609615633055,3.35954730743978));
#11506=CARTESIAN_POINT('',(-13.5433978507239,2.00000241142841,6.75365985713521));
#11507=CARTESIAN_POINT('',(-16.37182497547,2.00000241142841,3.92523273238902));
#11508=CARTESIAN_POINT('',(-19.7659375251655,2.00000241142841,0.531120182693588));
#11509=CARTESIAN_POINT('',(-13.5433978507239,-1.99999758857159,6.75365985713521));
#11510=CARTESIAN_POINT('',(-13.5433978507239,-3.53609615633055,6.75365985713521));
#11511=CARTESIAN_POINT('',(-16.37182497547,-1.99999758857159,3.92523273238902));
#11512=CARTESIAN_POINT('',(-19.7659375251655,-1.99999758857159,0.531120182693588));
#11513=CARTESIAN_POINT('',(-16.37182497547,-3.53609615633055,3.92523273238902));
#11514=CARTESIAN_POINT('',(-16.37182497547,2.00000241142841,3.92523273238902));
#11515=CARTESIAN_POINT('Origin',(-9.15718923943328,2.4114284077716E-6,-4.42077385354621));
#11516=CARTESIAN_POINT('',(-16.37182497547,2.00000241142841,2.79386188249054));
#11517=CARTESIAN_POINT('',(-15.1031958253685,2.00000241142841,1.52523273238902));
#11518=CARTESIAN_POINT('',(-9.15718923943328,2.00000241142841,-4.42077385354621));
#11519=CARTESIAN_POINT('',(-16.37182497547,3.53610097918737,2.79386188249054));
#11520=CARTESIAN_POINT('',(-15.1031958253685,2.00000241142841,1.52523273238902));
#11521=CARTESIAN_POINT('Origin',(-10.1492853010284,2.00000241142841,2.2281764575413));
#11522=CARTESIAN_POINT('',(-12.2747687006223,-1.99999758857159,4.35365985713521));
#11523=CARTESIAN_POINT('',(-13.5433978507238,-1.99999758857159,5.62228900723673));
#11524=CARTESIAN_POINT('',(-10.1492853010284,-1.99999758857159,2.2281764575413));
#11525=CARTESIAN_POINT('',(-13.5433978507238,2.00000241142841,5.62228900723673));
#11526=CARTESIAN_POINT('',(-13.5433978507238,2.00000241142841,5.62228900723673));
#11527=CARTESIAN_POINT('',(-12.2747687006223,2.00000241142841,4.35365985713521));
#11528=CARTESIAN_POINT('',(-10.1492853010284,2.00000241142841,2.2281764575413));
#11529=CARTESIAN_POINT('',(-12.2747687006223,2.00000241142841,4.35365985713521));
#11530=CARTESIAN_POINT('Origin',(-15.8061395505208,-1.99999758857159,-3.42867779195108));
#11531=CARTESIAN_POINT('Origin',(-15.8061395505208,-1.99999758857159,3.35954730743978));
#11532=CARTESIAN_POINT('Origin',(-12.9777124257746,-1.99999758857159,6.18797443218597));
#11533=CARTESIAN_POINT('Origin',(-11.7090832756731,-1.99999758857159,4.91934528208444));
#11534=CARTESIAN_POINT('Origin',(-14.5375104004193,-1.99999758857159,2.09091815733826));
#11535=CARTESIAN_POINT('Origin',(-15.8061395505208,2.00000241142841,-3.42867779195108));
#11536=CARTESIAN_POINT('Origin',(-15.8061395505208,2.00000241142841,3.35954730743978));
#11537=CARTESIAN_POINT('Origin',(-14.5375104004193,2.00000241142841,2.09091815733826));
#11538=CARTESIAN_POINT('Origin',(-11.7090832756731,2.00000241142841,4.91934528208444));
#11539=CARTESIAN_POINT('Origin',(-12.9777124257746,2.00000241142841,6.18797443218597));
#11540=CARTESIAN_POINT('Origin',(-14.6061395505208,-4.33609615633055,3.29091815733825));
#11541=CARTESIAN_POINT('Origin',(-14.6061395505208,4.33590384366945,3.29091815733825));
#11542=CARTESIAN_POINT('Origin',(-12.9777124257746,2.00000241142841,6.18797443218597));
#11543=CARTESIAN_POINT('Origin',(-15.8061395505208,2.4114284077716E-6,3.35954730743978));
#11544=CARTESIAN_POINT('Origin',(-15.8061395505208,2.4114284077716E-6,3.35954730743978));
#11545=CARTESIAN_POINT('Origin',(-14.5375104004193,2.4114284077716E-6,2.09091815733826));
#11546=CARTESIAN_POINT('Origin',(-14.5375104004193,2.4114284077716E-6,2.09091815733826));
#11547=CARTESIAN_POINT('Origin',(-11.7090832756731,3.53610097918737,4.91934528208444));
#11548=CARTESIAN_POINT('Origin',(-0.177712466787677,2.4114284077716E-6,
40.5587029190994));
#11549=CARTESIAN_POINT('',(-3.73255732111315,-3.53609615633055,40.5587029190994));
#11550=CARTESIAN_POINT('',(3.37713238753779,-3.53609615633055,40.5587029190994));
#11551=CARTESIAN_POINT('',(5.77713238753779,-3.53609615633055,40.5587029190994));
#11552=CARTESIAN_POINT('',(3.37713238753779,3.53610097918737,40.5587029190994));
#11553=CARTESIAN_POINT('',(3.37713238753779,3.53610097918737,40.5587029190994));
#11554=CARTESIAN_POINT('',(-3.73255732111315,3.53610097918737,40.5587029190994));
#11555=CARTESIAN_POINT('',(5.77713238753779,3.53610097918737,40.5587029190994));
#11556=CARTESIAN_POINT('',(-3.73255732111315,-3.53609615633055,40.5587029190994));
#11557=CARTESIAN_POINT('Origin',(5.77713238753779,-3.53609615633055,1.29011815733825));
#11558=CARTESIAN_POINT('',(5.77713238753779,-3.53609615633055,38.1587029190994));
#11559=CARTESIAN_POINT('',(5.77713238753779,-3.53609615633055,1.29011815733825));
#11560=CARTESIAN_POINT('Origin',(3.37713238753779,-3.53609615633055,38.1587029190994));
#11561=CARTESIAN_POINT('',(-6.13255732111315,-3.53609615633055,38.1587029190994));
#11562=CARTESIAN_POINT('Origin',(-3.73255732111315,-3.53609615633055,38.1587029190994));
#11563=CARTESIAN_POINT('',(-6.13255732111315,-3.53609615633055,1.29011815733825));
#11564=CARTESIAN_POINT('Origin',(5.77713238753779,3.53610097918737,1.29011815733825));
#11565=CARTESIAN_POINT('',(5.77713238753779,3.53610097918737,38.1587029190994));
#11566=CARTESIAN_POINT('',(5.77713238753779,3.53610097918737,1.29011815733825));
#11567=CARTESIAN_POINT('',(5.77713238753779,-3.53609615633055,38.1587029190994));
#11568=CARTESIAN_POINT('Origin',(5.77713238753779,3.53610097918737,1.29011815733825));
#11569=CARTESIAN_POINT('Origin',(3.37713238753779,3.53610097918737,38.1587029190994));
#11570=CARTESIAN_POINT('',(-6.13255732111315,3.53610097918737,38.1587029190994));
#11571=CARTESIAN_POINT('',(-6.13255732111315,3.53610097918737,1.29011815733825));
#11572=CARTESIAN_POINT('Origin',(-3.73255732111315,3.53610097918737,38.1587029190994));
#11573=CARTESIAN_POINT('Origin',(-6.13255732111315,3.53610097918737,1.29011815733825));
#11574=CARTESIAN_POINT('',(-6.13255732111315,3.53610097918737,38.1587029190994));
#11575=CARTESIAN_POINT('Origin',(3.37713238753779,2.4114284077716E-6,38.1587029190994));
#11576=CARTESIAN_POINT('Origin',(-3.73255732111315,2.4114284077716E-6,38.1587029190994));
#11577=CARTESIAN_POINT('Origin',(-4.21925722373829,20.,17.6406068922372));
#11578=CARTESIAN_POINT('Origin',(-4.21925722373829,20.,17.6406068922372));
#11579=CARTESIAN_POINT('Origin',(9.60397861284329,20.,11.8903072744979));
#11580=CARTESIAN_POINT('Origin',(9.60397861284329,20.,11.8903072744979));
#11581=CARTESIAN_POINT('',(6.42417721261744,20.,14.4149297172206));
#11582=CARTESIAN_POINT('Origin',(9.60397861284329,20.,11.8903072744979));
#11583=CARTESIAN_POINT('',(6.42417721261744,20.,14.4149297172206));
#11584=CARTESIAN_POINT('Origin',(-10.8056176096432,20.,28.0946289238114));
#11585=CARTESIAN_POINT('Origin',(-10.8056176096432,20.,28.0946289238114));
#13153=UNCERTAINTY_MEASURE_WITH_UNIT(LENGTH_MEASURE(0.01),#13200,
'DISTANCE_ACCURACY_VALUE',
'Maximum model space distance between geometric entities at asserted c
onnectivities');
#13173=UNCERTAINTY_MEASURE_WITH_UNIT(LENGTH_MEASURE(0.01),#13200,
'DISTANCE_ACCURACY_VALUE',
'Maximum model space distance between geometric entities at asserted c
onnectivities');
#13179=(
GEOMETRIC_REPRESENTATION_CONTEXT(3)
GLOBAL_UNCERTAINTY_ASSIGNED_CONTEXT((#13153))
GLOBAL_UNIT_ASSIGNED_CONTEXT((#13200,#13202,#13203))
REPRESENTATION_CONTEXT('','3D')
);
#13199=(
GEOMETRIC_REPRESENTATION_CONTEXT(3)
GLOBAL_UNCERTAINTY_ASSIGNED_CONTEXT((#13173))
GLOBAL_UNIT_ASSIGNED_CONTEXT((#13200,#13202,#13203))
REPRESENTATION_CONTEXT('','3D')
);
#13200=(
LENGTH_UNIT()
NAMED_UNIT(*)
SI_UNIT(.MILLI.,.METRE.)
);
#13202=(
NAMED_UNIT(*)
PLANE_ANGLE_UNIT()
SI_UNIT($,.RADIAN.)
);
#13203=(
NAMED_UNIT(*)
SI_UNIT($,.STERADIAN.)
SOLID_ANGLE_UNIT()
);
#13209=SHAPE_DEFINITION_REPRESENTATION(#13234,#13283);
#13234=PRODUCT_DEFINITION_SHAPE('',$,#13309);
#13283=SHAPE_REPRESENTATION('',(#7359),#13179);
#13303=PRODUCT_DEFINITION_CONTEXT('part definition',#13380,'design');
#13309=PRODUCT_DEFINITION('Finger Link 3','Finger Link 3',#13334,#13303);
#13334=PRODUCT_DEFINITION_FORMATION('',$,#13387);
#13380=APPLICATION_CONTEXT(
'Core Data for Automotive Mechanical Design Process');
#13381=PRODUCT_CONTEXT('part definition',#13380,'mechanical');
#13387=PRODUCT('Finger Link 3','Finger Link 3',$,(#13381));
#13409=PRESENTATION_STYLE_ASSIGNMENT((#13414));
#13414=SURFACE_STYLE_USAGE(.BOTH.,#13419);
#13419=SURFACE_SIDE_STYLE('',(#13424));
#13424=SURFACE_STYLE_FILL_AREA(#13429);
#13429=FILL_AREA_STYLE('Opaque(61,176,222)',(#13434));
#13434=FILL_AREA_STYLE_COLOUR('Opaque(61,176,222)',#13439);
#13439=COLOUR_RGB('Opaque(61,176,222)',0.23921568627451,0.690196078431373,
0.870588235294118);
ENDSEC;
END-ISO-10303-21;
